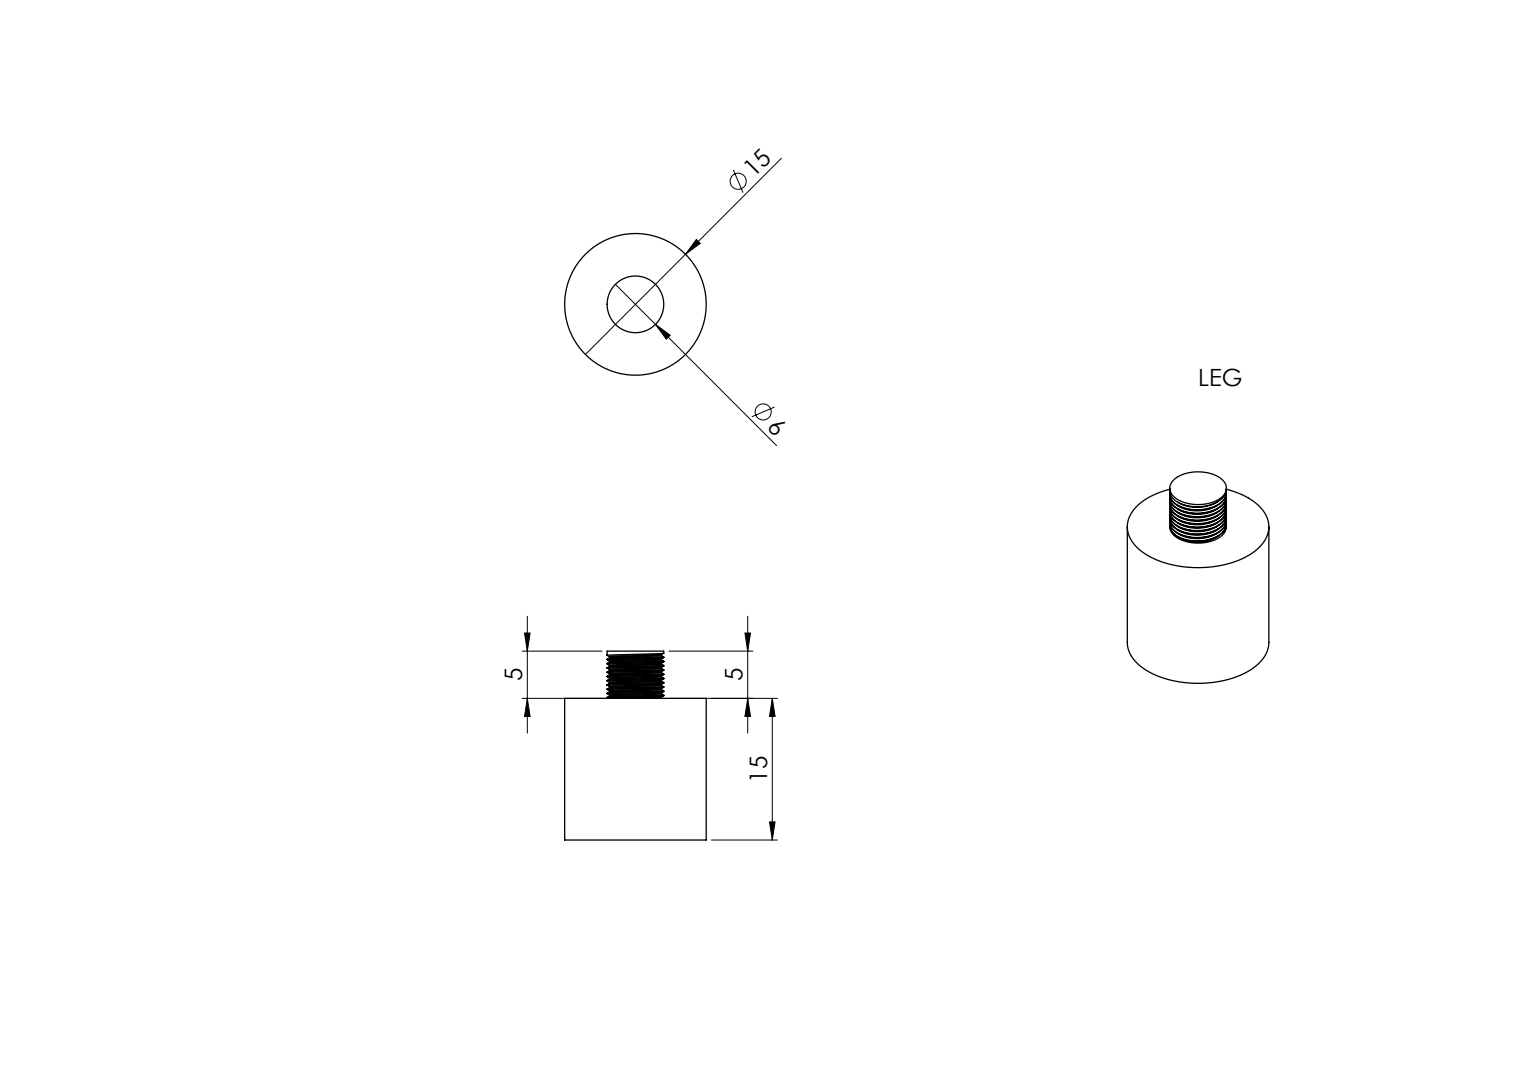
ISO-10303-21;
HEADER;
FILE_DESCRIPTION (('STEP AP214'),
    '1' );
FILE_NAME ('leg.step',
    '2026-10-25T17:17:34',
    ( '' ),
    ( '' ),
    'SwSTEP 2.0',
    'SolidWorks 2026',
    '' );
FILE_SCHEMA (( 'AUTOMOTIVE_DESIGN' ));
ENDSEC;

DATA;
#1=CARTESIAN_POINT ( 'NONE',  ( -79.64356964375001269, -33.59062499938548285, 98.40857419181659793 ) ) ;
#12=CARTESIAN_POINT ( 'NONE',  ( -82.39999999999999147, -34.07812499938548711, 103.1828516163667899 ) ) ;
#16=CARTESIAN_POINT ( 'NONE',  ( -85.39999999999999147, -34.97364041986484295, 98.90809577818235709 ) ) ;
#22=CARTESIAN_POINT ( 'NONE',  ( -79.39999999999999147, -33.41250000000000142, 101.7320508075688537 ) ) ;
#23=CARTESIAN_POINT ( 'NONE',  ( -83.90000000000000568, -30.46874999877096712, 97.40192378864668399 ) ) ;
#27=EDGE_CURVE ( 'NONE', #9630, #12897, #3914, .T. ) ;
#34=CARTESIAN_POINT ( 'NONE',  ( -85.15643035624999868, -31.00312499938548072, 101.5914258081833879 ) ) ;
#40=CARTESIAN_POINT ( 'NONE',  ( -85.40000000000000568, -31.38749999999999574, 98.26794919243111792 ) ) ;
#54=EDGE_CURVE ( 'NONE', #12568, #18235, #14634, .T. ) ;
#61=CARTESIAN_POINT ( 'NONE',  ( -79.39999999999999147, -31.03124999877097068, 98.26794919243110371 ) ) ;
#63=CARTESIAN_POINT ( 'NONE',  ( -85.40000000000000568, -31.38356250001228531, 98.26794919243111792 ) ) ;
#67=CARTESIAN_POINT ( 'NONE',  ( -85.15643035624999868, -31.97812499938548925, 98.40857419181659793 ) ) ;
#73=DIRECTION ( 'NONE',  ( -0.000000000000000000, -1.000000000000000000, -0.000000000000000000 ) ) ;
#93=CARTESIAN_POINT ( 'NONE',  ( -79.39999999999999147, -32.91018749875867400, 101.7320508075688537 ) ) ;
#95=CARTESIAN_POINT ( 'NONE',  ( -82.39999999999999147, -34.19062499938548427, 103.1828516163667899 ) ) ;
#109=CARTESIAN_POINT ( 'NONE',  ( -79.64356964374998427, -33.10312499938548569, 101.5914258081833879 ) ) ;
#112=ORIENTED_EDGE ( 'NONE', *, *, #10203, .F. ) ;
#115=CARTESIAN_POINT ( 'NONE',  ( -82.39999999999999147, -34.83749999999999858, 103.0000000000000000 ) ) ;
#121=CARTESIAN_POINT ( 'NONE',  ( -83.90000000000000568, -34.57500000000000284, 97.40192378864668399 ) ) ;
#122=CARTESIAN_POINT ( 'NONE',  ( -79.39999999999999147, -31.93124999877096926, 98.26794919243110371 ) ) ;
#132=CARTESIAN_POINT ( 'NONE',  ( -82.65380294351676582, -34.99990492518305274, 97.01075526832239859 ) ) ;
#135=CARTESIAN_POINT ( 'NONE',  ( -81.02178482187500208, -31.19062499938548427, 97.61286128772489690 ) ) ;
#141=CARTESIAN_POINT ( 'NONE',  ( -79.39999999999999147, -30.26249999999999929, 101.7320508075688537 ) ) ;
#149=ORIENTED_EDGE ( 'NONE', *, *, #9637, .F. ) ;
#160=CARTESIAN_POINT ( 'NONE',  ( -79.39999999999999147, -32.43356250001229313, 98.26794919243110371 ) ) ;
#189=CARTESIAN_POINT ( 'NONE',  ( -80.90000000000000568, -32.49768749875867968, 102.5980762113533018 ) ) ;
#190=CARTESIAN_POINT ( 'NONE',  ( -83.77821517812500929, -33.02812499938548285, 97.61286128772489690 ) ) ;
#203=CARTESIAN_POINT ( 'NONE',  ( -83.77821517812500929, -33.36562499938548854, 97.61286128772489690 ) ) ;
#204=EDGE_LOOP ( 'NONE', ( #12601, #4330, #15037, #10087 ) ) ;
#212=CARTESIAN_POINT ( 'NONE',  ( -85.40000000000000568, -30.35045094645306563, 101.9998975609119469 ) ) ;
#213=CARTESIAN_POINT ( 'NONE',  ( -82.39999999999999147, -30.73124999877096641, 103.4641016151377499 ) ) ;
#216=CARTESIAN_POINT ( 'NONE',  ( -82.39999999999999147, -35.09062499938548285, 103.1828516163667899 ) ) ;
#222=ORIENTED_EDGE ( 'NONE', *, *, #5417, .T. ) ;
#233=CARTESIAN_POINT ( 'NONE',  ( -83.90000000000000568, -30.07499999999999929, 97.40192378864668399 ) ) ;
#245=CARTESIAN_POINT ( 'NONE',  ( -80.90000000000000568, -31.59374999877097423, 102.5980762113533018 ) ) ;
#248=STYLED_ITEM ( 'NONE', ( #13866 ), #18578 ) ;
#250=CARTESIAN_POINT ( 'NONE',  ( -83.77821517812500929, -31.52812499938548996, 102.3871387122750889 ) ) ;
#254=CARTESIAN_POINT ( 'NONE',  ( -82.31848699153323423, -34.99951142137499716, 103.0191144166183221 ) ) ;
#259=CARTESIAN_POINT ( 'NONE',  ( -85.40000000000000568, -34.96970290221972277, 98.90809659374338025 ) ) ;
#262=CARTESIAN_POINT ( 'NONE',  ( -79.64356964374998427, -30.51562499938548711, 101.5914258081833879 ) ) ;
#276=VECTOR ( 'NONE', #14347, 1000.000000000000000 ) ;
#286=CARTESIAN_POINT ( 'NONE',  ( -79.39999999999999147, -31.52268749875867471, 99.99999999999998579 ) ) ;
#288=CARTESIAN_POINT ( 'NONE',  ( -82.39999999999999147, -33.74062499938548854, 103.1828516163667899 ) ) ;
#304=CARTESIAN_POINT ( 'NONE',  ( -85.15643035625001289, -35.05312499938548143, 101.5914258081833879 ) ) ;
#314=CARTESIAN_POINT ( 'NONE',  ( -79.39999999999999147, -33.78750000000000142, 98.26794919243110371 ) ) ;
#316=CARTESIAN_POINT ( 'NONE',  ( -83.90000000000000568, -30.91874999877096997, 97.40192378864668399 ) ) ;
#319=CARTESIAN_POINT ( 'NONE',  ( -79.39999999999999147, -30.71250000000000213, 101.7320508075688537 ) ) ;
#322=CARTESIAN_POINT ( 'NONE',  ( -82.40000000000000568, -30.00000000000000355, 103.0000000000000000 ) ) ;
#327=FILL_AREA_STYLE ('',( #7917 ) ) ;
#329=DIRECTION ( 'NONE',  ( -0.000000000000000000, -1.000000000000000000, -0.000000000000000000 ) ) ;
#353=CARTESIAN_POINT ( 'NONE',  ( -83.77821517812500929, -30.32812499938548711, 97.61286128772489690 ) ) ;
#357=CARTESIAN_POINT ( 'NONE',  ( -79.76502430829106061, -35.00019033771674515, 98.52379045060148144 ) ) ;
#361=CARTESIAN_POINT ( 'NONE',  ( -83.77821517812500929, -31.07812499938548711, 102.3871387122750889 ) ) ;
#371=CARTESIAN_POINT ( 'NONE',  ( -85.40000000000000568, -33.18750000000000000, 98.26794919243111792 ) ) ;
#380=CARTESIAN_POINT ( 'NONE',  ( -80.90000000000000568, -35.19768749875867542, 102.5980762113533018 ) ) ;
#408=CARTESIAN_POINT ( 'NONE',  ( -82.40000000000000568, -33.93750000000000711, 102.9999999999999858 ) ) ;
#409=CARTESIAN_POINT ( 'NONE',  ( -82.39999999999999147, -30.95624999877097139, 96.53589838486223584 ) ) ;
#410=CARTESIAN_POINT ( 'NONE',  ( -80.90000000000000568, -34.14374999877097139, 97.40192378864668399 ) ) ;
#414=CARTESIAN_POINT ( 'NONE',  ( -85.15643035625001289, -35.22676544108147567, 98.99674642581742035 ) ) ;
#418=ORIENTED_EDGE ( 'NONE', *, *, #10898, .T. ) ;
#441=ORIENTED_EDGE ( 'NONE', *, *, #8685, .F. ) ;
#446=CARTESIAN_POINT ( 'NONE',  ( -79.64356964375001269, -32.24062499938548854, 98.40857419181659793 ) ) ;
#450=CARTESIAN_POINT ( 'NONE',  ( -84.70833260042415702, -35.00006955123599539, 98.08383195543535749 ) ) ;
#454=CARTESIAN_POINT ( 'NONE',  ( -83.77821517812500929, -30.62812499938548783, 102.3871387122750889 ) ) ;
#467=DIRECTION ( 'NONE',  ( 0.000000000000000000, 0.000000000000000000, -1.000000000000000000 ) ) ;
#475=CARTESIAN_POINT ( 'NONE',  ( -85.40000000000000568, -34.03518749875867400, 98.26794919243111792 ) ) ;
#488=CARTESIAN_POINT ( 'NONE',  ( -82.39999999999999147, -33.85312499938547859, 96.81714838363319586 ) ) ;
#500=CARTESIAN_POINT ( 'NONE',  ( -82.39999999999999147, -31.40624999877097068, 96.53589838486223584 ) ) ;
#501=CARTESIAN_POINT ( 'NONE',  ( -82.39999999999999147, -33.20624999877097139, 96.53589838486223584 ) ) ;
#502=CARTESIAN_POINT ( 'NONE',  ( -82.40000000000000568, -30.50624999877097210, 96.99999999999998579 ) ) ;
#521=CARTESIAN_POINT ( 'NONE',  ( -85.40000000000000568, -30.39374999877097139, 99.99999999999998579 ) ) ;
#536=CARTESIAN_POINT ( 'NONE',  ( -79.64356964375001269, -31.41562499938548569, 101.5914258081833879 ) ) ;
#546=CARTESIAN_POINT ( 'NONE',  ( -83.77821517812500929, -32.57812499938548711, 97.61286128772489690 ) ) ;
#555=EDGE_CURVE ( 'NONE', #2812, #11515, #13893, .T. ) ;
#571=CARTESIAN_POINT ( 'NONE',  ( -80.90000000000000568, -34.74768749875867968, 102.5980762113533018 ) ) ;
#580=AXIS2_PLACEMENT_3D ( 'NONE', #9951, #8566, #14520 ) ;
#589=CARTESIAN_POINT ( 'NONE',  ( -83.77821517812500929, -32.31562499938548427, 102.3871387122750889 ) ) ;
#601=CARTESIAN_POINT ( 'NONE',  ( -82.40000000000001990, -32.13750000000000284, 103.0000000000000000 ) ) ;
#602=CARTESIAN_POINT ( 'NONE',  ( -85.40000000000000568, -31.33124999877096428, 98.26794919243111792 ) ) ;
#604=CARTESIAN_POINT ( 'NONE',  ( -79.39999999999999147, -35.11874999877096570, 99.99999999999998579 ) ) ;
#607=CARTESIAN_POINT ( 'NONE',  ( -82.40000000000000568, -30.50624999877097210, 96.99999999999998579 ) ) ;
#612=ORIENTED_EDGE ( 'NONE', *, *, #5825, .F. ) ;
#613=CARTESIAN_POINT ( 'NONE',  ( -83.90000000000000568, -33.46874999877096712, 102.5980762113533018 ) ) ;
#616=CYLINDRICAL_SURFACE ( 'NONE', #18162, 3.000000000000002665 ) ;
#619=CARTESIAN_POINT ( 'NONE',  ( -81.59615242270665192, -33.86115380933864571, 103.0000000000000000 ) ) ;
#625=CARTESIAN_POINT ( 'NONE',  ( -79.39999999999999147, -33.82106250001229597, 99.99999999999998579 ) ) ;
#632=EDGE_LOOP ( 'NONE', ( #11535, #18764, #13842, #12752 ) ) ;
#636=CARTESIAN_POINT ( 'NONE',  ( -83.20384757729335945, -30.80759618943233846, 102.9999999999999858 ) ) ;
#638=CARTESIAN_POINT ( 'NONE',  ( -83.77821517812500929, -31.97812499938548925, 102.3871387122750889 ) ) ;
#647=CARTESIAN_POINT ( 'NONE',  ( -81.02178482187500208, -31.30312499938548498, 97.61286128772489690 ) ) ;
#650=ADVANCED_FACE ( 'NONE', ( #8903 ), #14768, .T. ) ;
#667=ADVANCED_FACE ( 'NONE', ( #13111 ), #7348, .T. ) ;
#669=CARTESIAN_POINT ( 'NONE',  ( -79.39999999999999147, -34.71018749875867826, 101.7320508075688537 ) ) ;
#683=CARTESIAN_POINT ( 'NONE',  ( -83.77821517812500929, -34.56562499938548427, 102.3871387122750889 ) ) ;
#689=ORIENTED_EDGE ( 'NONE', *, *, #8646, .T. ) ;
#693=CARTESIAN_POINT ( 'NONE',  ( -79.39999999999999147, -34.31250000000000000, 101.7320508075688537 ) ) ;
#694=CARTESIAN_POINT ( 'NONE',  ( -79.39999999999999147, -32.90624999877096712, 101.7320508075688537 ) ) ;
#696=CARTESIAN_POINT ( 'NONE',  ( -85.40000000000000568, -34.03124999877096712, 98.26794919243111792 ) ) ;
#697=CARTESIAN_POINT ( 'NONE',  ( -83.90000000000000568, -32.17500000000000426, 102.5980762113533018 ) ) ;
#706=LINE ( 'NONE', #16822, #18035 ) ;
#710=CARTESIAN_POINT ( 'NONE',  ( -82.40000000000000568, -35.00000000000000000, 99.99999999999998579 ) ) ;
#712=CARTESIAN_POINT ( 'NONE',  ( -79.39999999999999147, -31.93124999877096926, 98.26794919243110371 ) ) ;
#714=CARTESIAN_POINT ( 'NONE',  ( -82.40000000000001990, -33.88124999877096855, 103.0000000000000000 ) ) ;
#716=( BOUNDED_CURVE ( )  B_SPLINE_CURVE ( 2, ( #8573, #10335, #8671, #13360, #14625, #1549, #11516, #4377, #5749 ),
 .UNSPECIFIED., .F., .F. ) 
 B_SPLINE_CURVE_WITH_KNOTS ( ( 3, 2, 2, 2, 3 ),
 ( 0.3125000000000001665, 0.3194444444444444198, 0.3333333333333333148, 0.3472222222222222099, 0.3541666666666666297 ),
 .UNSPECIFIED. ) 
 CURVE ( )  GEOMETRIC_REPRESENTATION_ITEM ( )  RATIONAL_B_SPLINE_CURVE ( ( 0.9330127018922194093, 0.9330127018922209636, 1.000000000000000000, 0.8660254037844387076, 1.000000000000000000, 0.8660254037844387076, 1.000000000000000000, 0.9330127018922196314, 0.9330127018922194093 ) ) 
 REPRESENTATION_ITEM ( '' )  );
#718=DIRECTION ( 'NONE',  ( -0.000000000000000000, -1.000000000000000000, -0.000000000000000000 ) ) ;
#720=CARTESIAN_POINT ( 'NONE',  ( -80.90000000000000568, -30.30000000000000426, 102.5980762113533018 ) ) ;
#724=DIRECTION ( 'NONE',  ( -0.000000000000000000, -1.000000000000000000, -0.000000000000000000 ) ) ;
#733=CARTESIAN_POINT ( 'NONE',  ( -82.39999999999999147, -33.06562499938548427, 96.81714838363319586 ) ) ;
#740=CARTESIAN_POINT ( 'NONE',  ( -81.02178482187500208, -32.65312499938548996, 97.61286128772489690 ) ) ;
#750=CARTESIAN_POINT ( 'NONE',  ( -83.20384757729335945, -33.00134618820329990, 102.9999999999999858 ) ) ;
#762=CARTESIAN_POINT ( 'NONE',  ( -79.39999999999999147, -33.36018749875868394, 101.7320508075688537 ) ) ;
#765=DIRECTION ( 'NONE',  ( 0.000000000000000000, -0.000000000000000000, 1.000000000000000000 ) ) ;
#767=FACE_OUTER_BOUND ( 'NONE', #5223, .T. ) ;
#776=CARTESIAN_POINT ( 'NONE',  ( -79.64356964374999848, -33.51562499938548711, 99.99999999999998579 ) ) ;
#788=CARTESIAN_POINT ( 'NONE',  ( -85.40000000000000568, -31.70624999877096784, 101.7320508075688679 ) ) ;
#789=CARTESIAN_POINT ( 'NONE',  ( -85.40000000000000568, -33.09374999877096712, 99.99999999999998579 ) ) ;
#805=CARTESIAN_POINT ( 'NONE',  ( -85.15643035625001289, -30.25312499938548783, 99.99999999999998579 ) ) ;
#806=STYLED_ITEM('',(#19357),#9467);
#811=CARTESIAN_POINT ( 'NONE',  ( -83.20384757729337366, -30.48615380933863150, 97.00000000000000000 ) ) ;
#813=CARTESIAN_POINT ( 'NONE',  ( -79.39999999999999147, -30.63750000000000284, 98.26794919243110371 ) ) ;
#828=CARTESIAN_POINT ( 'NONE',  ( -79.64356964375001269, -34.49062499938548854, 98.40857419181659793 ) ) ;
#837=CARTESIAN_POINT ( 'NONE',  ( -82.39999999999999147, -33.51562499938548711, 96.81714838363319586 ) ) ;
#846=CARTESIAN_POINT ( 'NONE',  ( -80.90000000000000568, -34.35000000000000853, 102.5980762113533018 ) ) ;
#853=CYLINDRICAL_SURFACE ( 'NONE', #4855, 3.000000000000002665 ) ;
#854=CARTESIAN_POINT ( 'NONE',  ( -85.40000000000000568, -30.48356250001229029, 98.26794919243111792 ) ) ;
#873=CARTESIAN_POINT ( 'NONE',  ( -79.64356964375001269, -33.10312499938549280, 101.5914258081833879 ) ) ;
#877=FACE_OUTER_BOUND ( 'NONE', #6470, .T. ) ;
#884=CARTESIAN_POINT ( 'NONE',  ( -82.39999999999999147, -31.63124999877097210, 103.4641016151377499 ) ) ;
#885=CARTESIAN_POINT ( 'NONE',  ( -85.40000000000000568, -35.36739044046696279, 98.90809476984486537 ) ) ;
#886=VECTOR ( 'NONE', #2876, 1000.000000000000000 ) ;
#897=ORIENTED_EDGE ( 'NONE', *, *, #8064, .F. ) ;
#899=CARTESIAN_POINT ( 'NONE',  ( -82.39999999999999147, -30.47812499938548569, 103.1828516163667899 ) ) ;
#905=ADVANCED_FACE ( 'NONE', ( #18104, #4715 ), #15646, .F. ) ;
#910=CARTESIAN_POINT ( 'NONE',  ( -83.90000000000000568, -33.97106250001230165, 102.5980762113533018 ) ) ;
#915=CYLINDRICAL_SURFACE ( 'NONE', #17436, 3.000000000000002665 ) ;
#917=( BOUNDED_CURVE ( )  B_SPLINE_CURVE ( 2, ( #8964, #4479, #7598, #11995, #3006, #16396, #4288, #14932, #1556 ),
 .UNSPECIFIED., .F., .F. ) 
 B_SPLINE_CURVE_WITH_KNOTS ( ( 3, 2, 2, 2, 3 ),
 ( 0.2708333333333333148, 0.2777777777777777901, 0.2916666666666666852, 0.3055555555555555802, 0.3125000000000001110 ),
 .UNSPECIFIED. ) 
 CURVE ( )  GEOMETRIC_REPRESENTATION_ITEM ( )  RATIONAL_B_SPLINE_CURVE ( ( 0.9330127018922194093, 0.9330127018922190762, 1.000000000000000000, 0.8660254037844387076, 1.000000000000000000, 0.8660254037844387076, 1.000000000000000000, 0.9330127018922182991, 0.9330127018922194093 ) ) 
 REPRESENTATION_ITEM ( '' )  );
#919=ORIENTED_EDGE ( 'NONE', *, *, #16886, .F. ) ;
#924=CARTESIAN_POINT ( 'NONE',  ( -79.64356964375001269, -35.01562499938548711, 101.5914258081833879 ) ) ;
#928=CARTESIAN_POINT ( 'NONE',  ( -82.30067660862302148, -35.00052948526250418, 96.98128288508057437 ) ) ;
#929=CARTESIAN_POINT ( 'NONE',  ( -85.15643035624999868, -34.67812499938548143, 98.40857419181659793 ) ) ;
#930=CARTESIAN_POINT ( 'NONE',  ( -82.40000000000000568, -35.00000000000000000, 107.5000000000000142 ) ) ;
#934=ADVANCED_FACE ( 'NONE', ( #12608 ), #616, .T. ) ;
#935=CARTESIAN_POINT ( 'NONE',  ( -79.64356964374998427, -34.56562499938548427, 101.5914258081833879 ) ) ;
#946=CARTESIAN_POINT ( 'NONE',  ( -80.90000000000000568, -33.45000000000000284, 102.5980762113533018 ) ) ;
#950=CARTESIAN_POINT ( 'NONE',  ( -83.90000000000000568, -31.42500000000000071, 97.40192378864668399 ) ) ;
#954=CARTESIAN_POINT ( 'NONE',  ( -82.40000000000000568, -30.00000000000000355, 99.99999999999998579 ) ) ;
#956=CARTESIAN_POINT ( 'NONE',  ( -85.40000000000000568, -30.93356250001229313, 98.26794919243111792 ) ) ;
#957=CYLINDRICAL_SURFACE ( 'NONE', #2043, 3.000000000000002665 ) ;
#959=CARTESIAN_POINT ( 'NONE',  ( -85.15643035625001289, -30.59062499938548285, 99.99999999999998579 ) ) ;
#960=DIRECTION ( 'NONE',  ( 0.000000000000000000, 0.000000000000000000, -1.000000000000000000 ) ) ;
#980=CARTESIAN_POINT ( 'NONE',  ( -80.90000000000000568, -34.74374999877097281, 102.5980762113533018 ) ) ;
#981=CARTESIAN_POINT ( 'NONE',  ( -85.15643035624999868, -31.56562499938548427, 101.5914258081833879 ) ) ;
#991=CARTESIAN_POINT ( 'NONE',  ( -83.90000000000000568, -35.26874999877097139, 102.5980762113533018 ) ) ;
#997=ORIENTED_EDGE ( 'NONE', *, *, #5541, .F. ) ;
#1004=CARTESIAN_POINT ( 'NONE',  ( -80.90000000000000568, -32.85000000000000142, 97.40192378864668399 ) ) ;
#1013=CARTESIAN_POINT ( 'NONE',  ( -82.40000000000000568, -30.00000000000000355, 96.99999999999998579 ) ) ;
#1019=CARTESIAN_POINT ( 'NONE',  ( -82.39999999999999147, -33.74062499938548854, 103.1828516163667899 ) ) ;
#1023=CARTESIAN_POINT ( 'NONE',  ( -83.77821517812500929, -34.26562499938548711, 97.61286128772489690 ) ) ;
#1028=CARTESIAN_POINT ( 'NONE',  ( -83.77821517812500929, -33.02812499938548285, 97.61286128772489690 ) ) ;
#1038=CARTESIAN_POINT ( 'NONE',  ( -83.90000000000000568, -33.22500000000000142, 97.40192378864668399 ) ) ;
#1039=AXIS2_PLACEMENT_3D ( 'NONE', #9542, #18538, #13936 ) ;
#1050=CARTESIAN_POINT ( 'NONE',  ( -79.64356964375001269, -30.32812499938548711, 98.40857419181659793 ) ) ;
#1059=CARTESIAN_POINT ( 'NONE',  ( -81.02178482187500208, -34.79062499938548569, 97.61286128772489690 ) ) ;
#1069=CARTESIAN_POINT ( 'NONE',  ( -82.39999999999999147, -35.23124999877096997, 103.4641016151377499 ) ) ;
#1070=CARTESIAN_POINT ( 'NONE',  ( -85.40000000000000568, -35.34374999877096712, 99.99999999999998579 ) ) ;
#1081=CARTESIAN_POINT ( 'NONE',  ( -85.15643035625001289, -31.49062499938548498, 99.99999999999998579 ) ) ;
#1089=CARTESIAN_POINT ( 'NONE',  ( -79.39999999999999147, -31.61250000000000071, 101.7320508075688537 ) ) ;
#1095=CARTESIAN_POINT ( 'NONE',  ( -79.39999999999999147, -31.08750000000000568, 98.26794919243110371 ) ) ;
#1102=CARTESIAN_POINT ( 'NONE',  ( -79.64356964375001269, -34.04062499938549280, 98.40857419181659793 ) ) ;
#1106=CARTESIAN_POINT ( 'NONE',  ( -82.39999999999999147, -33.85312499938547859, 96.81714838363319586 ) ) ;
#1114=CARTESIAN_POINT ( 'NONE',  ( -83.77821517812500929, -33.92812499938548854, 97.61286128772489690 ) ) ;
#1126=CARTESIAN_POINT ( 'NONE',  ( -80.90000000000000568, -34.20000000000000284, 97.40192378864668399 ) ) ;
#1148=ORIENTED_EDGE ( 'NONE', *, *, #9637, .T. ) ;
#1155=VERTEX_POINT ( 'NONE', #12694 ) ;
#1164=CARTESIAN_POINT ( 'NONE',  ( -83.90000000000000568, -33.61874999877097281, 97.40192378864668399 ) ) ;
#1166=CARTESIAN_POINT ( 'NONE',  ( -79.64356964374999848, -30.92812499938548498, 99.99999999999998579 ) ) ;
#1179=CARTESIAN_POINT ( 'NONE',  ( -79.64356964374998427, -31.30312499938548143, 101.5914258081833879 ) ) ;
#1180=VECTOR ( 'NONE', #3831, 1000.000000000000000 ) ;
#1187=CARTESIAN_POINT ( 'NONE',  ( -85.40000000000000568, -31.74374999877096926, 99.99999999999998579 ) ) ;
#1190=VECTOR ( 'NONE', #1364, 1000.000000000000000 ) ;
#1193=CARTESIAN_POINT ( 'NONE',  ( -82.39999999999999147, -32.13749999999999574, 103.4641016151377499 ) ) ;
#1202=CARTESIAN_POINT ( 'NONE',  ( -80.90000000000000568, -33.39374999877097139, 102.5980762113533018 ) ) ;
#1204=CARTESIAN_POINT ( 'NONE',  ( -82.39999999999999147, -31.60312499938548569, 96.81714838363319586 ) ) ;
#1208=CARTESIAN_POINT ( 'NONE',  ( -85.15643035624999868, -33.32812499938548001, 98.40857419181659793 ) ) ;
#1211=CARTESIAN_POINT ( 'NONE',  ( -82.40000000000000568, -30.00000000000000355, 103.0000000000000000 ) ) ;
#1215=CARTESIAN_POINT ( 'NONE',  ( -81.02178482187500208, -35.05312499938548854, 102.3871387122750889 ) ) ;
#1222=EDGE_LOOP ( 'NONE', ( #8619, #10140 ) ) ;
#1224=CARTESIAN_POINT ( 'NONE',  ( -82.40000000000000568, -30.00000000000000355, 99.99999999999998579 ) ) ;
#1226=CARTESIAN_POINT ( 'NONE',  ( -79.39999999999999147, -32.88750000000000284, 98.26794919243110371 ) ) ;
#1236=CARTESIAN_POINT ( 'NONE',  ( -82.40000000000000568, -30.00000000000000355, 96.99999999999998579 ) ) ;
#1238=CARTESIAN_POINT ( 'NONE',  ( -83.77821517812500929, -32.01562499938548001, 97.61286128772489690 ) ) ;
#1254=ORIENTED_EDGE ( 'NONE', *, *, #2671, .T. ) ;
#1265=CARTESIAN_POINT ( 'NONE',  ( -79.39999999999999147, -35.11874999877096570, 99.99999999999998579 ) ) ;
#1266=CARTESIAN_POINT ( 'NONE',  ( -81.02178482187500208, -31.75312499938548427, 97.61286128772489690 ) ) ;
#1272=VERTEX_POINT ( 'NONE', #607 ) ;
#1277=CARTESIAN_POINT ( 'NONE',  ( -83.77821517812500929, -32.91562499938547859, 97.61286128772489690 ) ) ;
#1290=CARTESIAN_POINT ( 'NONE',  ( -83.90000000000000568, -33.07500000000000284, 102.5980762113533018 ) ) ;
#1292=DIRECTION ( 'NONE',  ( 0.000000000000000000, 1.000000000000000000, 0.000000000000000000 ) ) ;
#1297=ORIENTED_EDGE ( 'NONE', *, *, #5113, .F. ) ;
#1303=CARTESIAN_POINT ( 'NONE',  ( -83.77821517812500929, -35.12812499938548427, 102.3871387122750889 ) ) ;
#1307=ORIENTED_EDGE ( 'NONE', *, *, #7912, .F. ) ;
#1309=CARTESIAN_POINT ( 'NONE',  ( -82.39999999999999147, -34.97812499938547859, 103.1828516163667899 ) ) ;
#1312=CARTESIAN_POINT ( 'NONE',  ( -83.90000000000000568, -32.62500000000000000, 102.5980762113533018 ) ) ;
#1317=VECTOR ( 'NONE', #9535, 1000.000000000000000 ) ;
#1328=EDGE_CURVE ( 'NONE', #7637, #16985, #16283, .T. ) ;
#1329=AXIS2_PLACEMENT_3D ( 'NONE', #5503, #1292, #12818 ) ;
#1331=( BOUNDED_CURVE ( )  B_SPLINE_CURVE ( 2, ( #6021, #10319, #7768, #12165, #6310, #16373, #13437, #7481, #15187 ),
 .UNSPECIFIED., .F., .F. ) 
 B_SPLINE_CURVE_WITH_KNOTS ( ( 3, 2, 2, 2, 3 ),
 ( 0.5208333333333333703, 0.5277777777777777901, 0.5416666666666666297, 0.5555555555555555802, 0.5625000000000000000 ),
 .UNSPECIFIED. ) 
 CURVE ( )  GEOMETRIC_REPRESENTATION_ITEM ( )  RATIONAL_B_SPLINE_CURVE ( ( 0.9330127018922192983, 0.9330127018922198534, 1.000000000000000000, 0.8660254037844387076, 1.000000000000000000, 0.8660254037844387076, 1.000000000000000000, 0.9330127018922194093, 0.9330127018922194093 ) ) 
 REPRESENTATION_ITEM ( '' )  );
#1334=CARTESIAN_POINT ( 'NONE',  ( -85.40000000000000568, -33.63356250001229597, 98.26794919243111792 ) ) ;
#1337=CARTESIAN_POINT ( 'NONE',  ( -85.15643035625001289, -31.94062499938548427, 99.99999999999998579 ) ) ;
#1361=CARTESIAN_POINT ( 'NONE',  ( -82.39999999999999147, -33.65624999877096712, 96.53589838486223584 ) ) ;
#1362=CARTESIAN_POINT ( 'NONE',  ( -81.02178482187500208, -32.80312499938548854, 102.3871387122750889 ) ) ;
#1364=DIRECTION ( 'NONE',  ( -0.000000000000000000, -1.000000000000000000, -0.000000000000000000 ) ) ;
#1365=ADVANCED_FACE ( 'NONE', ( #3175 ), #10413, .T. ) ;
#1375=CARTESIAN_POINT ( 'NONE',  ( -82.39999999999999147, -32.50312499938548427, 96.81714838363319586 ) ) ;
#1386=CARTESIAN_POINT ( 'NONE',  ( -85.40000000000000568, -32.70000000000000284, 99.99999999999998579 ) ) ;
#1387=CARTESIAN_POINT ( 'NONE',  ( -83.90000000000000568, -31.81874999877096855, 97.40192378864668399 ) ) ;
#1389=CARTESIAN_POINT ( 'NONE',  ( -84.69814161231457206, -35.29583579514545733, 98.07164704222797980 ) ) ;
#1395=CARTESIAN_POINT ( 'NONE',  ( -82.39999999999999147, -30.78750000000000142, 102.9999999999999858 ) ) ;
#1396=CARTESIAN_POINT ( 'NONE',  ( -82.39999999999999147, -30.92812499938548143, 103.1828516163667899 ) ) ;
#1402=CARTESIAN_POINT ( 'NONE',  ( -82.39999999999999147, -32.13749999999999574, 103.4641016151377499 ) ) ;
#1405=CARTESIAN_POINT ( 'NONE',  ( -82.40000000000001990, -31.68750000000000711, 103.0000000000000000 ) ) ;
#1418=( BOUNDED_CURVE ( )  B_SPLINE_CURVE ( 2, ( #15673, #15769, #12741, #7856, #9413, #12539, #15380, #16945, #18611 ),
 .UNSPECIFIED., .F., .F. ) 
 B_SPLINE_CURVE_WITH_KNOTS ( ( 3, 2, 2, 2, 3 ),
 ( 0.7708333333333331483, 0.7777777777777777901, 0.7916666666666666297, 0.8055555555555555802, 0.8125000000000001110 ),
 .UNSPECIFIED. ) 
 CURVE ( )  GEOMETRIC_REPRESENTATION_ITEM ( )  RATIONAL_B_SPLINE_CURVE ( ( 0.9330127018922194093, 0.9330127018922177440, 1.000000000000000000, 0.8660254037844387076, 1.000000000000000000, 0.8660254037844387076, 1.000000000000000000, 0.9330127018922182991, 0.9330127018922194093 ) ) 
 REPRESENTATION_ITEM ( '' )  );
#1424=CARTESIAN_POINT ( 'NONE',  ( -80.90000000000000568, -32.39606250001229881, 97.40192378864668399 ) ) ;
#1427=CARTESIAN_POINT ( 'NONE',  ( -79.64356964374999848, -32.16562499938548569, 99.99999999999998579 ) ) ;
#1450=CARTESIAN_POINT ( 'NONE',  ( -80.90000000000000568, -31.59768749875868110, 102.5980762113533018 ) ) ;
#1451=CARTESIAN_POINT ( 'NONE',  ( -85.15643035625001289, -32.50312499938548427, 99.99999999999998579 ) ) ;
#1455=CARTESIAN_POINT ( 'NONE',  ( -84.51155153715826884, -35.14114847181267720, 98.22820474807231506 ) ) ;
#1463=CARTESIAN_POINT ( 'NONE',  ( -82.39999999999999147, -33.85312499938548569, 96.81714838363319586 ) ) ;
#1474=CARTESIAN_POINT ( 'NONE',  ( -80.90000000000000568, -30.69374999877097210, 102.5980762113533018 ) ) ;
#1475=CARTESIAN_POINT ( 'NONE',  ( -82.39999999999999147, -30.50624999877097210, 96.53589838486223584 ) ) ;
#1491=CARTESIAN_POINT ( 'NONE',  ( -79.64356964375001269, -32.20312499938548001, 101.5914258081833879 ) ) ;
#1492=DIRECTION ( 'NONE',  ( 0.000000000000000000, -1.000000000000000000, 0.000000000000000000 ) ) ;
#1496=ORIENTED_EDGE ( 'NONE', *, *, #6126, .T. ) ;
#1499=CARTESIAN_POINT ( 'NONE',  ( -85.40000000000000568, -32.25000000000000000, 99.99999999999998579 ) ) ;
#1511=EDGE_CURVE ( 'NONE', #2507, #16323, #4665, .T. ) ;
#1524=CARTESIAN_POINT ( 'NONE',  ( -82.40000000000000568, -30.95624999877097139, 96.99999999999998579 ) ) ;
#1526=CARTESIAN_POINT ( 'NONE',  ( -83.90000000000000568, -32.77106250001229171, 97.40192378864668399 ) ) ;
#1530=CARTESIAN_POINT ( 'NONE',  ( -79.64356964375001269, -30.85312499938548569, 101.5914258081833879 ) ) ;
#1535=DIRECTION ( 'NONE',  ( 0.000000000000000000, 0.000000000000000000, -1.000000000000000000 ) ) ;
#1538=( BOUNDED_CURVE ( )  B_SPLINE_CURVE ( 2, ( #16992, #4802, #3314, #13857, #15532, #12495, #13768, #9271, #408 ),
 .UNSPECIFIED., .F., .F. ) 
 B_SPLINE_CURVE_WITH_KNOTS ( ( 3, 2, 2, 2, 3 ),
 ( 0.6875000000000000000, 0.6944444444444444198, 0.7083333333333333703, 0.7222222222222222099, 0.7291666666666668517 ),
 .UNSPECIFIED. ) 
 CURVE ( )  GEOMETRIC_REPRESENTATION_ITEM ( )  RATIONAL_B_SPLINE_CURVE ( ( 0.9330127018922194093, 0.9330127018922194093, 1.000000000000000000, 0.8660254037844387076, 1.000000000000000000, 0.8660254037844387076, 1.000000000000000000, 0.9330127018922177440, 0.9330127018922194093 ) ) 
 REPRESENTATION_ITEM ( '' )  );
#1549=CARTESIAN_POINT ( 'NONE',  ( -85.40000000000000568, -32.23124999877096997, 98.26794919243111792 ) ) ;
#1554=CARTESIAN_POINT ( 'NONE',  ( -79.39999999999999147, -31.48518749875868394, 98.26794919243110371 ) ) ;
#1555=CARTESIAN_POINT ( 'NONE',  ( -83.77821517812500929, -32.87812499938548427, 102.3871387122750889 ) ) ;
#1556=CARTESIAN_POINT ( 'NONE',  ( -82.40000000000000568, -31.68750000000000711, 102.9999999999999858 ) ) ;
#1567=CARTESIAN_POINT ( 'NONE',  ( -81.02178482187500208, -34.49062499938548854, 102.3871387122750889 ) ) ;
#1571=CARTESIAN_POINT ( 'NONE',  ( -82.40000000000000568, -34.10624999877096997, 96.99999999999998579 ) ) ;
#1577=CARTESIAN_POINT ( 'NONE',  ( -79.39999999999999147, -34.68750000000000000, 98.26794919243110371 ) ) ;
#1578=CARTESIAN_POINT ( 'NONE',  ( -79.39999999999999147, -32.41874999877096997, 99.99999999999998579 ) ) ;
#1589=CARTESIAN_POINT ( 'NONE',  ( -82.39999999999999147, -31.15312499938548640, 96.81714838363319586 ) ) ;
#1595=ORIENTED_EDGE ( 'NONE', *, *, #7912, .T. ) ;
#1597=CARTESIAN_POINT ( 'NONE',  ( -85.40000000000000568, -30.86250000000000071, 101.7320508075688679 ) ) ;
#1612=CARTESIAN_POINT ( 'NONE',  ( -83.32052461991715120, -34.98323688327303671, 97.06736352196708140 ) ) ;
#1615=ORIENTED_EDGE ( 'NONE', *, *, #11751, .T. ) ;
#1619=CARTESIAN_POINT ( 'NONE',  ( -85.40000000000000568, -31.83356250001229881, 98.26794919243111792 ) ) ;
#1625=DIRECTION ( 'NONE',  ( 0.000000000000000000, 0.000000000000000000, -1.000000000000000000 ) ) ;
#1627=ORIENTED_EDGE ( 'NONE', *, *, #11751, .F. ) ;
#1643=CARTESIAN_POINT ( 'NONE',  ( -83.90000000000000568, -33.02268749875867826, 102.5980762113533018 ) ) ;
#1644=CARTESIAN_POINT ( 'NONE',  ( -79.64356964374999848, -33.17812499938548854, 99.99999999999998579 ) ) ;
#1658=CARTESIAN_POINT ( 'NONE',  ( -85.15643035625001289, -33.29062499938547859, 99.99999999999998579 ) ) ;
#1663=CARTESIAN_POINT ( 'NONE',  ( -85.40000000000000568, -34.95000000000000284, 99.99999999999998579 ) ) ;
#1669=CARTESIAN_POINT ( 'NONE',  ( -85.40000000000000568, -34.05000000000000426, 99.99999999999998579 ) ) ;
#1670=CARTESIAN_POINT ( 'NONE',  ( -83.90000000000000568, -32.71874999877096712, 97.40192378864668399 ) ) ;
#1671=CARTESIAN_POINT ( 'NONE',  ( -82.40000000000000568, -30.00000000000000355, 99.99999999999998579 ) ) ;
#1687=CARTESIAN_POINT ( 'NONE',  ( -79.39999999999999147, -30.18750000000000355, 98.26794919243110371 ) ) ;
#1704=CARTESIAN_POINT ( 'NONE',  ( -84.94178044275902550, -34.99917348188823496, 101.6311593377337203 ) ) ;
#1707=CARTESIAN_POINT ( 'NONE',  ( -80.90000000000000568, -33.29606250001229739, 97.40192378864668399 ) ) ;
#1709=CARTESIAN_POINT ( 'NONE',  ( -79.64356964374999848, -31.82812499938548356, 99.99999999999998579 ) ) ;
#1731=CARTESIAN_POINT ( 'NONE',  ( -85.40000000000000568, -31.33518749875867471, 98.26794919243111792 ) ) ;
#1733=CARTESIAN_POINT ( 'NONE',  ( -83.77821517812500929, -33.47812499938548569, 97.61286128772489690 ) ) ;
#1755=DIRECTION ( 'NONE',  ( -0.000000000000000000, -1.000000000000000000, -0.000000000000000000 ) ) ;
#1758=CARTESIAN_POINT ( 'NONE',  ( -79.39999999999999147, -34.31250000000000000, 101.7320508075688537 ) ) ;
#1760=CARTESIAN_POINT ( 'NONE',  ( -80.90000000000000568, -31.44374999877096855, 97.40192378864668399 ) ) ;
#1787=ORIENTED_EDGE ( 'NONE', *, *, #2182, .F. ) ;
#1793=CARTESIAN_POINT ( 'NONE',  ( -81.02178482187500208, -32.20312499938548711, 97.61286128772489690 ) ) ;
#1797=CARTESIAN_POINT ( 'NONE',  ( -79.39923258946704721, -35.00058613678730524, 99.84651357762385260 ) ) ;
#1798=CARTESIAN_POINT ( 'NONE',  ( -80.90000000000000568, -31.14374999877097139, 102.5980762113533018 ) ) ;
#1803=CARTESIAN_POINT ( 'NONE',  ( -85.15643035625001289, -30.66562499938548569, 101.5914258081833879 ) ) ;
#1807=AXIS2_PLACEMENT_3D ( 'NONE', #10995, #6415, #6609 ) ;
#1813=CARTESIAN_POINT ( 'NONE',  ( -83.90000000000000568, -33.01874999877097139, 102.5980762113533018 ) ) ;
#1815=ADVANCED_FACE ( 'NONE', ( #16069 ), #2580, .T. ) ;
#1816=DIRECTION ( 'NONE',  ( 0.000000000000000000, 0.000000000000000000, -1.000000000000000000 ) ) ;
#1819=ORIENTED_EDGE ( 'NONE', *, *, #7074, .F. ) ;
#1828=CARTESIAN_POINT ( 'NONE',  ( -83.90000000000000568, -31.82268749875867542, 97.40192378864668399 ) ) ;
#1845=CARTESIAN_POINT ( 'NONE',  ( -85.15643035625001289, -35.09062499938548285, 99.99999999999998579 ) ) ;
#1846=ORIENTED_EDGE ( 'NONE', *, *, #7551, .F. ) ;
#1855=CARTESIAN_POINT ( 'NONE',  ( -83.90000000000000568, -33.97500000000000853, 102.5980762113533018 ) ) ;
#1856=CARTESIAN_POINT ( 'NONE',  ( -79.39999999999999147, -34.66874999877096997, 99.99999999999998579 ) ) ;
#1857=CARTESIAN_POINT ( 'NONE',  ( -81.59615242270662350, -30.52634618820330914, 97.00000000000000000 ) ) ;
#1858=CARTESIAN_POINT ( 'NONE',  ( -79.39999999999999147, -30.67500000000000071, 99.99999999999998579 ) ) ;
#1863=ORIENTED_EDGE ( 'NONE', *, *, #14991, .T. ) ;
#1864=( NAMED_UNIT ( * ) PLANE_ANGLE_UNIT ( ) SI_UNIT ( $, .RADIAN. ) );
#1889=CARTESIAN_POINT ( 'NONE',  ( -83.90000000000000568, -33.91874999877096997, 102.5980762113533018 ) ) ;
#1891=CARTESIAN_POINT ( 'NONE',  ( -83.77821517812500929, -30.62812499938548783, 102.3871387122750889 ) ) ;
#1895=CARTESIAN_POINT ( 'NONE',  ( -83.35106844018336858, -35.00071516271440686, 102.8502752770200601 ) ) ;
#1897=CARTESIAN_POINT ( 'NONE',  ( -81.59615242270662350, -32.56740381056766864, 103.0000000000000000 ) ) ;
#1899=CARTESIAN_POINT ( 'NONE',  ( -83.77821517812500929, -32.42812499938548854, 102.3871387122750889 ) ) ;
#1919=CARTESIAN_POINT ( 'NONE',  ( -85.40000000000000568, -33.96018749875868536, 101.7320508075688679 ) ) ;
#1936=CARTESIAN_POINT ( 'NONE',  ( -79.64356964375001269, -34.00312499938549138, 101.5914258081833879 ) ) ;
#1949=CARTESIAN_POINT ( 'NONE',  ( -80.90000000000000568, -32.79374999877096997, 97.40192378864668399 ) ) ;
#1950=( BOUNDED_CURVE ( )  B_SPLINE_CURVE ( 2, ( #5196, #14451, #9585, #712, #9979, #17110, #8312, #2349, #4017 ),
 .UNSPECIFIED., .F., .F. ) 
 B_SPLINE_CURVE_WITH_KNOTS ( ( 3, 2, 2, 2, 3 ),
 ( 0.2708333333333333703, 0.2777777777777777901, 0.2916666666666666852, 0.3055555555555555802, 0.3125000000000001665 ),
 .UNSPECIFIED. ) 
 CURVE ( )  GEOMETRIC_REPRESENTATION_ITEM ( )  RATIONAL_B_SPLINE_CURVE ( ( 0.9330127018922194093, 0.9330127018922196314, 1.000000000000000000, 0.8660254037844387076, 1.000000000000000000, 0.8660254037844387076, 1.000000000000000000, 0.9330127018922177440, 0.9330127018922194093 ) ) 
 REPRESENTATION_ITEM ( '' )  );
#1951=CARTESIAN_POINT ( 'NONE',  ( -79.39999999999999147, -33.35624999877097707, 101.7320508075688537 ) ) ;
#1952=CARTESIAN_POINT ( 'NONE',  ( -83.20384757729337366, -32.15759618943233278, 103.0000000000000000 ) ) ;
#1989=CARTESIAN_POINT ( 'NONE',  ( -83.77821517812500929, -31.22812499938548569, 97.61286128772489690 ) ) ;
#1994=CARTESIAN_POINT ( 'NONE',  ( -84.50041942204053669, -34.99839409658486034, 102.1701536479666999 ) ) ;
#1998=CARTESIAN_POINT ( 'NONE',  ( -81.02178482187500208, -30.85312499938548569, 97.61286128772489690 ) ) ;
#2009=CARTESIAN_POINT ( 'NONE',  ( -82.39999999999999147, -33.48750000000000426, 103.0000000000000000 ) ) ;
#2014=CARTESIAN_POINT ( 'NONE',  ( -79.39999999999999147, -32.83124999877097139, 98.26794919243110371 ) ) ;
#2016=CARTESIAN_POINT ( 'NONE',  ( -82.39999999999999147, -34.33518749875868536, 103.4641016151377499 ) ) ;
#2032=CARTESIAN_POINT ( 'NONE',  ( -79.64356964374999848, -33.06562499938548427, 99.99999999999998579 ) ) ;
#2034=VERTEX_POINT ( 'NONE', #18121 ) ;
#2037=CARTESIAN_POINT ( 'NONE',  ( -85.40000000000000568, -30.80624999877096570, 101.7320508075688821 ) ) ;
#2043=AXIS2_PLACEMENT_3D ( 'NONE', #5454, #6912, #18832 ) ;
#2045=CARTESIAN_POINT ( 'NONE',  ( -85.40000000000000568, -33.05624999877096570, 101.7320508075688679 ) ) ;
#2046=CARTESIAN_POINT ( 'NONE',  ( -82.39999999999999147, -35.00624999877097565, 96.53589838486223584 ) ) ;
#2057=CARTESIAN_POINT ( 'NONE',  ( -83.20384757729335945, -33.45134618820330985, 102.9999999999999858 ) ) ;
#2058=CARTESIAN_POINT ( 'NONE',  ( -85.40000000000000568, -30.39374999877097139, 99.99999999999998579 ) ) ;
#2071=CARTESIAN_POINT ( 'NONE',  ( -85.40000000000000568, -34.00856250001229597, 101.7320508075688679 ) ) ;
#2086=CARTESIAN_POINT ( 'NONE',  ( -85.15643035625001289, -30.70312499938548711, 99.99999999999998579 ) ) ;
#2090=ORIENTED_EDGE ( 'NONE', *, *, #7559, .F. ) ;
#2095=CARTESIAN_POINT ( 'NONE',  ( -85.15643035625001289, -30.70312499938548711, 99.99999999999998579 ) ) ;
#2114=AXIS2_PLACEMENT_3D ( 'NONE', #19302, #11861, #16360 ) ;
#2120=CARTESIAN_POINT ( 'NONE',  ( -82.39999999999999147, -34.56018749875867258, 96.53589838486223584 ) ) ;
#2135=SHAPE_DEFINITION_REPRESENTATION ( #13860, #16991 ) ;
#2138=CARTESIAN_POINT ( 'NONE',  ( -79.64356964375001269, -34.45312499938548711, 101.5914258081833879 ) ) ;
#2150=CARTESIAN_POINT ( 'NONE',  ( -79.39999999999999147, -31.48124999877097352, 98.26794919243110371 ) ) ;
#2151=CARTESIAN_POINT ( 'NONE',  ( -85.40000000000000568, -33.50624999877096855, 101.7320508075688679 ) ) ;
#2173=CARTESIAN_POINT ( 'NONE',  ( -82.39999999999999147, -30.11250000000000426, 96.53589838486223584 ) ) ;
#2182=EDGE_CURVE ( 'NONE', #18235, #10587, #17387, .T. ) ;
#2186=CARTESIAN_POINT ( 'NONE',  ( -85.15643035624999868, -30.29062499938548925, 98.40857419181659793 ) ) ;
#2194=CARTESIAN_POINT ( 'NONE',  ( -83.77821517812500929, -34.37812499938548427, 97.61286128772489690 ) ) ;
#2213=CARTESIAN_POINT ( 'NONE',  ( -83.90000000000000568, -35.27268749875867826, 102.5980762113533018 ) ) ;
#2215=CARTESIAN_POINT ( 'NONE',  ( -79.64356964375001269, -35.01562499938548711, 101.5914258081833879 ) ) ;
#2226=CARTESIAN_POINT ( 'NONE',  ( -82.39999999999999147, -32.50312499938548427, 96.81714838363319586 ) ) ;
#2229=EDGE_CURVE ( 'NONE', #4020, #14453, #5179, .T. ) ;
#2232=ORIENTED_EDGE ( 'NONE', *, *, #8150, .T. ) ;
#2237=CARTESIAN_POINT ( 'NONE',  ( -82.39999999999999147, -33.20624999877097139, 96.53589838486223584 ) ) ;
#2238=CARTESIAN_POINT ( 'NONE',  ( -80.90000000000000568, -34.29374999877096997, 102.5980762113533018 ) ) ;
#2255=CARTESIAN_POINT ( 'NONE',  ( -79.39999999999999147, -33.73124999877096997, 98.26794919243110371 ) ) ;
#2261=CARTESIAN_POINT ( 'NONE',  ( -79.39999999999999147, -34.75856250001229597, 101.7320508075688537 ) ) ;
#2269=( BOUNDED_CURVE ( )  B_SPLINE_CURVE ( 2, ( #115, #7422, #13382, #16414, #1663, #16, #4494 ),
 .UNSPECIFIED., .F., .F. ) 
 B_SPLINE_CURVE_WITH_KNOTS ( ( 3, 2, 2, 3 ),
 ( 0.8958333333333333703, 0.9027777777777777901, 0.9166666666666666297, 0.9258785066912882389 ),
 .UNSPECIFIED. ) 
 CURVE ( )  GEOMETRIC_REPRESENTATION_ITEM ( )  RATIONAL_B_SPLINE_CURVE ( ( 0.9330127018922192983, 0.9330127018922198534, 1.000000000000000000, 0.8660254037844387076, 1.000000000000000000, 0.9111410165655264848, 0.9401539157124900736 ) ) 
 REPRESENTATION_ITEM ( '' )  );
#2277=CARTESIAN_POINT ( 'NONE',  ( -81.02178482187500208, -34.90312499938548285, 97.61286128772489690 ) ) ;
#2279=EDGE_LOOP ( 'NONE', ( #4183, #10015, #9450, #7227 ) ) ;
#2286=CARTESIAN_POINT ( 'NONE',  ( -83.77821517812500929, -32.87812499938548427, 102.3871387122750889 ) ) ;
#2294=CARTESIAN_POINT ( 'NONE',  ( -79.39999999999999147, -33.82500000000000284, 99.99999999999998579 ) ) ;
#2302=DIRECTION ( 'NONE',  ( -0.000000000000000000, -1.000000000000000000, -0.000000000000000000 ) ) ;
#2303=CARTESIAN_POINT ( 'NONE',  ( -79.39999999999999147, -30.70856250001229526, 101.7320508075688537 ) ) ;
#2305=CARTESIAN_POINT ( 'NONE',  ( -85.40000000000000568, -33.58518749875867826, 98.26794919243111792 ) ) ;
#2321=CARTESIAN_POINT ( 'NONE',  ( -81.02178482187500208, -33.59062499938548285, 102.3871387122750889 ) ) ;
#2327=VERTEX_POINT ( 'NONE', #11554 ) ;
#2332=CARTESIAN_POINT ( 'NONE',  ( -79.39999999999999147, -33.35624999877097707, 101.7320508075688537 ) ) ;
#2333=CARTESIAN_POINT ( 'NONE',  ( -81.02178482187500208, -31.00312499938548783, 102.3871387122750889 ) ) ;
#2334=CARTESIAN_POINT ( 'NONE',  ( -82.40000000000000568, -30.73124999877097352, 102.9999999999999858 ) ) ;
#2347=CARTESIAN_POINT ( 'NONE',  ( -85.15643035625001289, -30.62812499938548427, 98.40857419181659793 ) ) ;
#2349=CARTESIAN_POINT ( 'NONE',  ( -81.59615242270662350, -32.06115380933863435, 103.0000000000000000 ) ) ;
#2354=EDGE_CURVE ( 'NONE', #15766, #19154, #11162, .T. ) ;
#2357=CARTESIAN_POINT ( 'NONE',  ( -79.39999999999999147, -30.18750000000000355, 98.26794919243110371 ) ) ;
#2361=EDGE_CURVE ( 'NONE', #15766, #19060, #5321, .T. ) ;
#2368=CARTESIAN_POINT ( 'NONE',  ( -82.40000000000001990, -33.20624999877097849, 97.00000000000000000 ) ) ;
#2371=CARTESIAN_POINT ( 'NONE',  ( -79.64356964375001269, -34.56562499938549138, 101.5914258081833879 ) ) ;
#2376=CARTESIAN_POINT ( 'NONE',  ( -82.39999999999999147, -34.52812499938548996, 103.1828516163667899 ) ) ;
#2382=CARTESIAN_POINT ( 'NONE',  ( -85.15643035625001289, -34.26562499938548711, 101.5914258081833879 ) ) ;
#2393=CARTESIAN_POINT ( 'NONE',  ( -80.90000000000000568, -32.40000000000000568, 97.40192378864668399 ) ) ;
#2403=FACE_OUTER_BOUND ( 'NONE', #17857, .T. ) ;
#2404=CARTESIAN_POINT ( 'NONE',  ( -81.02178482187500208, -30.44062499938548783, 102.3871387122750889 ) ) ;
#2419=( GEOMETRIC_REPRESENTATION_CONTEXT ( 3 ) GLOBAL_UNCERTAINTY_ASSIGNED_CONTEXT ( ( #18388 ) ) GLOBAL_UNIT_ASSIGNED_CONTEXT ( ( #5002, #1864, #15640 ) ) REPRESENTATION_CONTEXT ( 'NONE', 'WORKASPACE' ) );
#2432=CARTESIAN_POINT ( 'NONE',  ( -80.90000000000000568, -33.39374999877097139, 102.5980762113533018 ) ) ;
#2433=CARTESIAN_POINT ( 'NONE',  ( -79.64356964375001269, -32.24062499938548854, 98.40857419181659793 ) ) ;
#2436=CIRCLE ( 'NONE', #17096, 7.500000000000020428 ) ;
#2448=CARTESIAN_POINT ( 'NONE',  ( -79.39999999999999147, -35.11874999877096570, 99.99999999999998579 ) ) ;
#2449=CARTESIAN_POINT ( 'NONE',  ( -82.39999999999999147, -30.70312499938548711, 96.81714838363319586 ) ) ;
#2451=ORIENTED_EDGE ( 'NONE', *, *, #12261, .F. ) ;
#2454=CARTESIAN_POINT ( 'NONE',  ( -80.90000000000000568, -33.69374999877096855, 97.40192378864668399 ) ) ;
#2459=CARTESIAN_POINT ( 'NONE',  ( -82.39999999999999147, -34.83356250001229171, 103.4641016151377499 ) ) ;
#2463=CARTESIAN_POINT ( 'NONE',  ( -79.39999999999999147, -33.41250000000000142, 101.7320508075688537 ) ) ;
#2465=CARTESIAN_POINT ( 'NONE',  ( -81.59615242270662350, -31.21740381056766722, 103.0000000000000000 ) ) ;
#2471=CARTESIAN_POINT ( 'NONE',  ( -81.02178482187500208, -33.25312499938548427, 102.3871387122750889 ) ) ;
#2473=ORIENTED_EDGE ( 'NONE', *, *, #6390, .T. ) ;
#2475=CARTESIAN_POINT ( 'NONE',  ( -81.02178482187500208, -34.04062499938548569, 102.3871387122750889 ) ) ;
#2479=CARTESIAN_POINT ( 'NONE',  ( -82.39999999999999147, -34.86562499938548854, 96.81714838363319586 ) ) ;
#2489=CARTESIAN_POINT ( 'NONE',  ( -85.15643035625001289, -30.14062499938548711, 99.99999999999998579 ) ) ;
#2490=CARTESIAN_POINT ( 'NONE',  ( -85.40000000000000568, -32.66250000000000142, 101.7320508075688679 ) ) ;
#2495=FACE_OUTER_BOUND ( 'NONE', #6682, .T. ) ;
#2496=CARTESIAN_POINT ( 'NONE',  ( -79.39999999999999147, -31.08356250001229171, 98.26794919243110371 ) ) ;
#2499=CARTESIAN_POINT ( 'NONE',  ( -81.02178482187500208, -30.74062499938548498, 97.61286128772489690 ) ) ;
#2507=VERTEX_POINT ( 'NONE', #10467 ) ;
#2511=CARTESIAN_POINT ( 'NONE',  ( -81.02178482187500208, -34.94062499938548427, 102.3871387122750889 ) ) ;
#2515=DIRECTION ( 'NONE',  ( -0.000000000000000000, -1.000000000000000000, -0.000000000000000000 ) ) ;
#2521=CARTESIAN_POINT ( 'NONE',  ( -84.69814161231455785, -35.39427329483935836, 98.07164704222793716 ) ) ;
#2522=CARTESIAN_POINT ( 'NONE',  ( -79.64356964374999848, -31.37812499938548427, 99.99999999999998579 ) ) ;
#2532=CARTESIAN_POINT ( 'NONE',  ( -82.39999999999999147, -30.92812499938548143, 103.1828516163667899 ) ) ;
#2543=CARTESIAN_POINT ( 'NONE',  ( -80.90000000000000568, -32.10000000000000142, 102.5980762113533018 ) ) ;
#2550=VERTEX_POINT ( 'NONE', #10284 ) ;
#2553=VECTOR ( 'NONE', #2515, 1000.000000000000000 ) ;
#2557=CARTESIAN_POINT ( 'NONE',  ( -83.77821517812500929, -32.87812499938548427, 102.3871387122750889 ) ) ;
#2562=CARTESIAN_POINT ( 'NONE',  ( -81.02178482187500208, -33.89062499938548711, 97.61286128772489690 ) ) ;
#2563=EDGE_CURVE ( 'NONE', #11976, #6642, #13389, .T. ) ;
#2571=CARTESIAN_POINT ( 'NONE',  ( -79.64356964374998427, -33.59062499938548285, 98.40857419181659793 ) ) ;
#2580=CYLINDRICAL_SURFACE ( 'NONE', #8809, 3.000000000000002665 ) ;
#2582=CARTESIAN_POINT ( 'NONE',  ( -82.39999999999999147, -32.81250000000000000, 96.53589838486223584 ) ) ;
#2586=DIRECTION ( 'NONE',  ( -0.000000000000000000, -1.000000000000000000, -0.000000000000000000 ) ) ;
#2593=CARTESIAN_POINT ( 'NONE',  ( -83.77821517812500929, -30.21562499938548285, 97.61286128772489690 ) ) ;
#2600=ORIENTED_EDGE ( 'NONE', *, *, #13152, .F. ) ;
#2605=( BOUNDED_CURVE ( )  B_SPLINE_CURVE ( 1, ( #1455, #6243 ),
 .UNSPECIFIED., .F., .F. ) 
 B_SPLINE_CURVE_WITH_KNOTS ( ( 2, 2 ),
 ( 0.000000000000000000, 1.000000000000000000 ),
 .UNSPECIFIED. ) 
 CURVE ( )  GEOMETRIC_REPRESENTATION_ITEM ( )  RATIONAL_B_SPLINE_CURVE ( ( 0.9401542295229963209, 0.9401542295229963209 ) ) 
 REPRESENTATION_ITEM ( '' )  );
#2616=CARTESIAN_POINT ( 'NONE',  ( -82.39999999999999147, -30.51018749875868252, 96.53589838486223584 ) ) ;
#2617=CARTESIAN_POINT ( 'NONE',  ( -79.64356964375001269, -31.79062499938548569, 98.40857419181659793 ) ) ;
#2627=CARTESIAN_POINT ( 'NONE',  ( -82.39999999999999147, -31.82812499938548356, 103.1828516163667899 ) ) ;
#2638=CARTESIAN_POINT ( 'NONE',  ( -79.39999999999999147, -31.08750000000000213, 98.26794919243110371 ) ) ;
#2649=AXIS2_PLACEMENT_3D ( 'NONE', #7712, #1755, #9366 ) ;
#2653=CARTESIAN_POINT ( 'NONE',  ( -79.64356964374999848, -30.81562499938548427, 99.99999999999998579 ) ) ;
#2659=CARTESIAN_POINT ( 'NONE',  ( -82.39999999999999147, -33.40312499938548285, 96.81714838363319586 ) ) ;
#2671=EDGE_CURVE ( 'NONE', #19154, #12568, #4037, .T. ) ;
#2679=CARTESIAN_POINT ( 'NONE',  ( -83.90000000000000568, -32.62500000000000000, 102.5980762113533018 ) ) ;
#2687=CARTESIAN_POINT ( 'NONE',  ( -82.39999999999999147, -30.10856250001229384, 96.53589838486223584 ) ) ;
#2689=CARTESIAN_POINT ( 'NONE',  ( -82.39999999999999147, -34.83749999999999858, 103.0000000000000000 ) ) ;
#2692=CARTESIAN_POINT ( 'NONE',  ( -83.90000000000000568, -32.56874999877096855, 102.5980762113533018 ) ) ;
#2707=ORIENTED_EDGE ( 'NONE', *, *, #8266, .T. ) ;
#2713=ADVANCED_FACE ( 'NONE', ( #15547 ), #15346, .T. ) ;
#2717=CARTESIAN_POINT ( 'NONE',  ( -83.90000000000000568, -30.47268749875867755, 97.40192378864668399 ) ) ;
#2719=CARTESIAN_POINT ( 'NONE',  ( -81.02178482187500208, -31.30312499938548498, 97.61286128772489690 ) ) ;
#2731=CARTESIAN_POINT ( 'NONE',  ( -81.02178482187500208, -30.29062499938548569, 97.61286128772489690 ) ) ;
#2739=CARTESIAN_POINT ( 'NONE',  ( -82.39999999999999147, -31.85624999877096641, 96.99999999999998579 ) ) ;
#2744=CARTESIAN_POINT ( 'NONE',  ( -79.39999999999999147, -32.92500000000000426, 99.99999999999998579 ) ) ;
#2757=CARTESIAN_POINT ( 'NONE',  ( -79.39999999999999147, -33.28124999877096712, 98.26794919243110371 ) ) ;
#2759=CARTESIAN_POINT ( 'NONE',  ( -83.77821517812500929, -31.56562499938548427, 97.61286128772489690 ) ) ;
#2765=CARTESIAN_POINT ( 'NONE',  ( -85.15643035624999868, -33.25312499938548427, 101.5914258081833879 ) ) ;
#2781=DIRECTION ( 'NONE',  ( -0.000000000000000000, -1.000000000000000000, -0.000000000000000000 ) ) ;
#2784=( BOUNDED_CURVE ( )  B_SPLINE_CURVE ( 2, ( #7473, #16463, #11676, #7184, #11581, #4255, #17544, #10214, #2787 ),
 .UNSPECIFIED., .F., .F. ) 
 B_SPLINE_CURVE_WITH_KNOTS ( ( 3, 2, 2, 2, 3 ),
 ( 0.06250000000000002776, 0.06944444444444444753, 0.08333333333333332871, 0.09722222222222222376, 0.1041666666666666713 ),
 .UNSPECIFIED. ) 
 CURVE ( )  GEOMETRIC_REPRESENTATION_ITEM ( )  RATIONAL_B_SPLINE_CURVE ( ( 0.9330127018922194093, 0.9330127018922196314, 1.000000000000000000, 0.8660254037844387076, 1.000000000000000000, 0.8660254037844387076, 1.000000000000000000, 0.9330127018922192983, 0.9330127018922194093 ) ) 
 REPRESENTATION_ITEM ( '' )  );
#2787=CARTESIAN_POINT ( 'NONE',  ( -82.40000000000000568, -30.56250000000001066, 96.99999999999998579 ) ) ;
#2789=ADVANCED_FACE ( 'NONE', ( #9287 ), #15444, .T. ) ;
#2792=CARTESIAN_POINT ( 'NONE',  ( -83.90000000000000568, -31.72106250001229810, 102.5980762113533018 ) ) ;
#2795=CARTESIAN_POINT ( 'NONE',  ( -79.64356964374999848, -30.81562499938548427, 99.99999999999998579 ) ) ;
#2812=VERTEX_POINT ( 'NONE', #4814 ) ;
#2818=CARTESIAN_POINT ( 'NONE',  ( -83.90000000000000568, -33.46874999877096712, 102.5980762113533018 ) ) ;
#2819=CARTESIAN_POINT ( 'NONE',  ( -85.15643035624999868, -34.34062499938548285, 98.40857419181659793 ) ) ;
#2831=CARTESIAN_POINT ( 'NONE',  ( -85.15643035625001289, -34.22812499938548569, 98.40857419181659793 ) ) ;
#2841=CARTESIAN_POINT ( 'NONE',  ( -85.40000000000000568, -31.83750000000000568, 98.26794919243111792 ) ) ;
#2846=CARTESIAN_POINT ( 'NONE',  ( -84.69814099439363986, -35.09873396208577390, 98.07164630581206666 ) ) ;
#2852=CYLINDRICAL_SURFACE ( 'NONE', #16778, 3.000000000000002665 ) ;
#2855=CARTESIAN_POINT ( 'NONE',  ( -81.02178482187500208, -35.05312499938548854, 102.3871387122750889 ) ) ;
#2861=CARTESIAN_POINT ( 'NONE',  ( -80.90000000000000568, -32.10000000000000142, 102.5980762113533018 ) ) ;
#2868=AXIS2_PLACEMENT_3D ( 'NONE', #18269, #13954, #9665 ) ;
#2876=DIRECTION ( 'NONE',  ( -0.000000000000000000, -1.000000000000000000, -0.000000000000000000 ) ) ;
#2885=CARTESIAN_POINT ( 'NONE',  ( -82.39999999999999147, -32.58356250001229881, 103.4641016151377499 ) ) ;
#2888=CARTESIAN_POINT ( 'NONE',  ( -83.77821517812500929, -30.96562499938548640, 102.3871387122750889 ) ) ;
#2907=CARTESIAN_POINT ( 'NONE',  ( -79.39999999999999147, -30.26250000000000284, 101.7320508075688537 ) ) ;
#2913=CARTESIAN_POINT ( 'NONE',  ( -85.40000000000000568, -32.61018749875868394, 101.7320508075688679 ) ) ;
#2914=CARTESIAN_POINT ( 'NONE',  ( -79.64356964375001269, -32.76562499938548711, 101.5914258081833879 ) ) ;
#2921=ORIENTED_EDGE ( 'NONE', *, *, #8685, .T. ) ;
#2926=CARTESIAN_POINT ( 'NONE',  ( -79.64356964374999848, -33.96562499938548285, 99.99999999999998579 ) ) ;
#2936=CARTESIAN_POINT ( 'NONE',  ( -82.39999999999999147, -33.71249999999999858, 96.53589838486223584 ) ) ;
#2937=EDGE_CURVE ( 'NONE', #3433, #6642, #16534, .T. ) ;
#2938=CARTESIAN_POINT ( 'NONE',  ( -80.90000000000000568, -30.99374999877096926, 97.40192378864668399 ) ) ;
#2939=CARTESIAN_POINT ( 'NONE',  ( -82.40000000000000568, -30.00000000000000355, 99.99999999999998579 ) ) ;
#2946=CARTESIAN_POINT ( 'NONE',  ( -84.51155386534844638, -35.25364837475780888, 98.22820752270799005 ) ) ;
#2948=CARTESIAN_POINT ( 'NONE',  ( -79.64356964374999848, -32.16562499938548569, 99.99999999999998579 ) ) ;
#2950=EDGE_CURVE ( 'NONE', #3433, #6725, #4244, .T. ) ;
#2955=CARTESIAN_POINT ( 'NONE',  ( -83.90000000000000568, -30.97500000000000142, 97.40192378864668399 ) ) ;
#2970=CARTESIAN_POINT ( 'NONE',  ( -85.40000000000000568, -34.93124999877096570, 98.26794919243111792 ) ) ;
#2977=CARTESIAN_POINT ( 'NONE',  ( -79.39999999999999147, -32.47106250001229455, 99.99999999999998579 ) ) ;
#2980=CARTESIAN_POINT ( 'NONE',  ( -83.77821517812500929, -32.46562499938548285, 97.61286128772489690 ) ) ;
#3004=CARTESIAN_POINT ( 'NONE',  ( -83.90000000000000568, -31.67268749875867684, 102.5980762113533018 ) ) ;
#3005=CARTESIAN_POINT ( 'NONE',  ( -85.15643035624999868, -32.54062499938548569, 98.40857419181659793 ) ) ;
#3006=CARTESIAN_POINT ( 'NONE',  ( -79.39999999999999147, -31.57499999999999929, 99.99999999999998579 ) ) ;
#3013=ADVANCED_FACE ( 'NONE', ( #16671 ), #11981, .T. ) ;
#3018=CARTESIAN_POINT ( 'NONE',  ( -81.02178482187500208, -33.14062499938548711, 102.3871387122750889 ) ) ;
#3024=ORIENTED_EDGE ( 'NONE', *, *, #18429, .T. ) ;
#3028=EDGE_CURVE ( 'NONE', #14891, #19060, #15384, .T. ) ;
#3030=CARTESIAN_POINT ( 'NONE',  ( -79.39999999999999147, -34.72500000000000142, 99.99999999999998579 ) ) ;
#3032=CARTESIAN_POINT ( 'NONE',  ( -79.39999999999999147, -31.03124999877097068, 98.26794919243110371 ) ) ;
#3044=CARTESIAN_POINT ( 'NONE',  ( -79.64356964374999848, -31.71562499938548285, 99.99999999999998579 ) ) ;
#3051=CARTESIAN_POINT ( 'NONE',  ( -82.39999999999999147, -31.91250000000000497, 96.53589838486223584 ) ) ;
#3058=CARTESIAN_POINT ( 'NONE',  ( -82.40000000000001990, -33.88124999877096855, 103.0000000000000000 ) ) ;
#3067=CARTESIAN_POINT ( 'NONE',  ( -79.39999999999999147, -34.72500000000000142, 99.99999999999998579 ) ) ;
#3073=CARTESIAN_POINT ( 'NONE',  ( -82.40000000000000568, -34.10624999877096997, 96.99999999999998579 ) ) ;
#3074=CARTESIAN_POINT ( 'NONE',  ( -85.40000000000000568, -31.34606250001229810, 99.99999999999998579 ) ) ;
#3077=CARTESIAN_POINT ( 'NONE',  ( -85.15643035624999868, -31.45312499938548356, 101.5914258081833879 ) ) ;
#3098=CARTESIAN_POINT ( 'NONE',  ( -80.90000000000000568, -32.94768749875867542, 102.5980762113533018 ) ) ;
#3100=CARTESIAN_POINT ( 'NONE',  ( -85.15643035624999868, -34.79062499938548569, 98.40857419181659793 ) ) ;
#3105=CARTESIAN_POINT ( 'NONE',  ( -82.40000000000000568, -30.00000000000000355, 103.0000000000000000 ) ) ;
#3112=CARTESIAN_POINT ( 'NONE',  ( -79.64356964374999848, -32.61562499938548854, 99.99999999999998579 ) ) ;
#3114=ORIENTED_EDGE ( 'NONE', *, *, #18600, .F. ) ;
#3118=ORIENTED_EDGE ( 'NONE', *, *, #5910, .T. ) ;
#3119=CARTESIAN_POINT ( 'NONE',  ( -82.40000000000000568, -50.00000000000000000, 92.49999999999997158 ) ) ;
#3123=CARTESIAN_POINT ( 'NONE',  ( -80.90000000000000568, -30.54374999877096997, 97.40192378864668399 ) ) ;
#3124=CARTESIAN_POINT ( 'NONE',  ( -85.40000000000000568, -30.84374999877096712, 99.99999999999998579 ) ) ;
#3131=SURFACE_STYLE_USAGE ( .BOTH. , #18189 ) ;
#3136=CARTESIAN_POINT ( 'NONE',  ( -79.64356964375001269, -33.47812499938547859, 98.40857419181659793 ) ) ;
#3142=CARTESIAN_POINT ( 'NONE',  ( -83.90000000000000568, -30.52500000000000213, 97.40192378864668399 ) ) ;
#3163=CARTESIAN_POINT ( 'NONE',  ( -83.18600968418431307, -35.00069049296057955, 102.9003918199492915 ) ) ;
#3168=CARTESIAN_POINT ( 'NONE',  ( -82.39999999999999147, -31.90856250001229810, 96.53589838486223584 ) ) ;
#3175=FACE_OUTER_BOUND ( 'NONE', #9076, .T. ) ;
#3179=DIRECTION ( 'NONE',  ( 0.000000000000000000, 0.000000000000000000, -1.000000000000000000 ) ) ;
#3181=CARTESIAN_POINT ( 'NONE',  ( -83.20384757729335945, -33.05759618943233136, 102.9999999999999858 ) ) ;
#3186=EDGE_CURVE ( 'NONE', #12568, #1155, #11648, .T. ) ;
#3193=CARTESIAN_POINT ( 'NONE',  ( -79.39999999999999147, -30.66018749875867755, 101.7320508075688537 ) ) ;
#3195=CARTESIAN_POINT ( 'NONE',  ( -85.15643035624999868, -33.89062499938548711, 98.40857419181659793 ) ) ;
#3209=CARTESIAN_POINT ( 'NONE',  ( -79.64356964374998427, -34.00312499938548427, 101.5914258081833879 ) ) ;
#3216=ORIENTED_EDGE ( 'NONE', *, *, #2563, .T. ) ;
#3217=CARTESIAN_POINT ( 'NONE',  ( -83.90000000000000568, -31.36874999877096926, 97.40192378864668399 ) ) ;
#3220=CARTESIAN_POINT ( 'NONE',  ( -82.39999999999999147, -34.16250000000000142, 96.53589838486223584 ) ) ;
#3221=CARTESIAN_POINT ( 'NONE',  ( -85.40000000000000568, -31.25624999877096855, 101.7320508075688679 ) ) ;
#3222=FACE_OUTER_BOUND ( 'NONE', #204, .T. ) ;
#3239=CARTESIAN_POINT ( 'NONE',  ( -85.40000000000000568, -31.83750000000000568, 98.26794919243111792 ) ) ;
#3247=ORIENTED_EDGE ( 'NONE', *, *, #17486, .T. ) ;
#3254=CARTESIAN_POINT ( 'NONE',  ( -85.15643035624999868, -32.09062499938548996, 98.40857419181659793 ) ) ;
#3258=CARTESIAN_POINT ( 'NONE',  ( -79.43507259642450435, -35.00111651776678201, 99.51279508880003277 ) ) ;
#3260=CARTESIAN_POINT ( 'NONE',  ( -80.90000000000000568, -32.55000000000000426, 102.5980762113533018 ) ) ;
#3261=CARTESIAN_POINT ( 'NONE',  ( -82.39999999999999147, -34.38356250001228176, 103.4641016151377499 ) ) ;
#3265=CARTESIAN_POINT ( 'NONE',  ( -79.64356964374998427, -31.86562499938548143, 101.5914258081833879 ) ) ;
#3280=FACE_OUTER_BOUND ( 'NONE', #14173, .T. ) ;
#3288=CARTESIAN_POINT ( 'NONE',  ( -85.40000000000000568, -31.26018749875867186, 101.7320508075688679 ) ) ;
#3289=CARTESIAN_POINT ( 'NONE',  ( -84.51155386534844638, -35.25364837475780888, 98.22820752270799005 ) ) ;
#3296=ADVANCED_FACE ( 'NONE', ( #10089 ), #14377, .T. ) ;
#3304=CARTESIAN_POINT ( 'NONE',  ( -83.77821517812500929, -35.01562499938548711, 102.3871387122750889 ) ) ;
#3309=AXIS2_PLACEMENT_3D ( 'NONE', #14269, #718, #13985 ) ;
#3314=CARTESIAN_POINT ( 'NONE',  ( -80.90000000000000568, -33.75000000000000000, 97.40192378864668399 ) ) ;
#3315=CARTESIAN_POINT ( 'NONE',  ( -83.90000000000000568, -34.12500000000000000, 97.40192378864668399 ) ) ;
#3317=CARTESIAN_POINT ( 'NONE',  ( -80.90000000000000568, -33.39374999877097139, 102.5980762113533018 ) ) ;
#3331=CARTESIAN_POINT ( 'NONE',  ( -80.90000000000000568, -30.15000000000000213, 97.40192378864668399 ) ) ;
#3345=ADVANCED_FACE ( 'NONE', ( #17903 ), #2852, .T. ) ;
#3355=CARTESIAN_POINT ( 'NONE',  ( -79.64356964375001269, -30.51562499938548711, 101.5914258081833879 ) ) ;
#3358=ORIENTED_EDGE ( 'NONE', *, *, #4450, .T. ) ;
#3368=CARTESIAN_POINT ( 'NONE',  ( -79.64356964374998427, -30.89062499938548711, 98.40857419181659793 ) ) ;
#3392=CARTESIAN_POINT ( 'NONE',  ( -85.40000000000000568, -33.09768749875867400, 99.99999999999998579 ) ) ;
#3406=CARTESIAN_POINT ( 'NONE',  ( -81.02178482187500208, -34.94062499938548427, 102.3871387122750889 ) ) ;
#3408=EDGE_LOOP ( 'NONE', ( #5079, #441, #8494, #13671 ) ) ;
#3410=( BOUNDED_CURVE ( )  B_SPLINE_CURVE ( 2, ( #1524, #11866, #17834, #61, #18224, #6015, #1798, #9126, #11961 ),
 .UNSPECIFIED., .F., .F. ) 
 B_SPLINE_CURVE_WITH_KNOTS ( ( 3, 2, 2, 2, 3 ),
 ( 0.1041666666666666713, 0.1111111111111111049, 0.1250000000000000000, 0.1388888888888888951, 0.1458333333333334814 ),
 .UNSPECIFIED. ) 
 CURVE ( )  GEOMETRIC_REPRESENTATION_ITEM ( )  RATIONAL_B_SPLINE_CURVE ( ( 0.9330127018922194093, 0.9330127018922194093, 1.000000000000000000, 0.8660254037844387076, 1.000000000000000000, 0.8660254037844387076, 1.000000000000000000, 0.9330127018922180770, 0.9330127018922194093 ) ) 
 REPRESENTATION_ITEM ( '' )  );
#3416=CARTESIAN_POINT ( 'NONE',  ( -82.39999999999999147, -34.16250000000000142, 97.00000000000000000 ) ) ;
#3417=CARTESIAN_POINT ( 'NONE',  ( -80.90000000000000568, -31.59374999877097423, 102.5980762113533018 ) ) ;
#3418=CARTESIAN_POINT ( 'NONE',  ( -82.39999999999999147, -33.43124999877097281, 103.4641016151377499 ) ) ;
#3433=VERTEX_POINT ( 'NONE', #132 ) ;
#3437=( BOUNDED_CURVE ( )  B_SPLINE_CURVE ( 2, ( #11845, #17813, #10190, #7256, #10577, #17720, #8907, #12037, #4623 ),
 .UNSPECIFIED., .F., .F. ) 
 B_SPLINE_CURVE_WITH_KNOTS ( ( 3, 2, 2, 2, 3 ),
 ( 0.3125000000000001110, 0.3194444444444444198, 0.3333333333333333148, 0.3472222222222222099, 0.3541666666666666852 ),
 .UNSPECIFIED. ) 
 CURVE ( )  GEOMETRIC_REPRESENTATION_ITEM ( )  RATIONAL_B_SPLINE_CURVE ( ( 0.9330127018922194093, 0.9330127018922204085, 1.000000000000000000, 0.8660254037844387076, 1.000000000000000000, 0.8660254037844387076, 1.000000000000000000, 0.9330127018922190762, 0.9330127018922194093 ) ) 
 REPRESENTATION_ITEM ( '' )  );
#3442=CARTESIAN_POINT ( 'NONE',  ( -82.40000000000000568, -30.00000000000000355, 103.0000000000000000 ) ) ;
#3451=CARTESIAN_POINT ( 'NONE',  ( -83.77821517812500929, -32.57812499938548711, 97.61286128772489690 ) ) ;
#3459=CARTESIAN_POINT ( 'NONE',  ( -79.64356964374998427, -30.96562499938548640, 101.5914258081833879 ) ) ;
#3480=CARTESIAN_POINT ( 'NONE',  ( -83.90000000000000568, -33.17268749875866973, 97.40192378864668399 ) ) ;
#3483=CARTESIAN_POINT ( 'NONE',  ( -85.40000000000000568, -34.44374999877096855, 99.99999999999998579 ) ) ;
#3497=CARTESIAN_POINT ( 'NONE',  ( -85.15643035625001289, -32.39062499938548711, 99.99999999999998579 ) ) ;
#3499=ORIENTED_EDGE ( 'NONE', *, *, #9854, .T. ) ;
#3502=CARTESIAN_POINT ( 'NONE',  ( -83.90000000000000568, -30.91874999877096997, 97.40192378864668399 ) ) ;
#3510=CARTESIAN_POINT ( 'NONE',  ( -85.40000000000000568, -31.25624999877096855, 101.7320508075688679 ) ) ;
#3511=CARTESIAN_POINT ( 'NONE',  ( -80.90000000000000568, -33.84374999877096712, 102.5980762113533018 ) ) ;
#3523=( BOUNDED_CURVE ( )  B_SPLINE_CURVE ( 2, ( #4770, #3768, #9436, #3576, #8363, #10905, #9735, #5147, #9642 ),
 .UNSPECIFIED., .F., .F. ) 
 B_SPLINE_CURVE_WITH_KNOTS ( ( 3, 2, 2, 2, 3 ),
 ( 0.3541666666666666297, 0.3611111111111111049, 0.3750000000000000000, 0.3888888888888888951, 0.3958333333333334259 ),
 .UNSPECIFIED. ) 
 CURVE ( )  GEOMETRIC_REPRESENTATION_ITEM ( )  RATIONAL_B_SPLINE_CURVE ( ( 0.9330127018922194093, 0.9330127018922190762, 1.000000000000000000, 0.8660254037844387076, 1.000000000000000000, 0.8660254037844387076, 1.000000000000000000, 0.9330127018922185211, 0.9330127018922192983 ) ) 
 REPRESENTATION_ITEM ( '' )  );
#3526=CLOSED_SHELL ( 'NONE', ( #5779, #17132, #6134, #11799, #1815, #10200, #17470, #1365, #19082, #4921, #3013, #6402, #15074, #16330, #934, #7816, #3296, #10940, #3345, #18227, #18400, #9723, #17020, #2713, #650, #905, #12213, #2789, #10924, #11662, #667, #8417, #17025, #13751 ) ) ;
#3542=CARTESIAN_POINT ( 'NONE',  ( -80.90000000000000568, -33.30000000000000426, 97.40192378864668399 ) ) ;
#3545=ORIENTED_EDGE ( 'NONE', *, *, #8064, .T. ) ;
#3549=CARTESIAN_POINT ( 'NONE',  ( -85.40000000000000568, -34.03124999877096712, 98.26794919243111792 ) ) ;
#3551=CARTESIAN_POINT ( 'NONE',  ( -79.64356964374999848, -31.37812499938548427, 99.99999999999998579 ) ) ;
#3554=EDGE_LOOP ( 'NONE', ( #6738, #7388, #9688, #4859 ) ) ;
#3560=CARTESIAN_POINT ( 'NONE',  ( -85.15643035625001289, -31.56562499938548427, 101.5914258081833879 ) ) ;
#3576=CARTESIAN_POINT ( 'NONE',  ( -79.39999999999999147, -32.38124999877096855, 98.26794919243110371 ) ) ;
#3579=CARTESIAN_POINT ( 'NONE',  ( -79.39999999999999147, -35.08518749875868536, 98.26794919243110371 ) ) ;
#3582=CARTESIAN_POINT ( 'NONE',  ( -81.02178482187500208, -35.05312499938548854, 102.3871387122750889 ) ) ;
#3583=CARTESIAN_POINT ( 'NONE',  ( -85.40000000000000568, -34.48124999877096997, 98.26794919243111792 ) ) ;
#3594=CARTESIAN_POINT ( 'NONE',  ( -81.02178482187500208, -34.34062499938548285, 97.61286128772489690 ) ) ;
#3604=LINE ( 'NONE', #12308, #12554 ) ;
#3605=CARTESIAN_POINT ( 'NONE',  ( -82.39999999999999147, -32.75624999877096855, 96.53589838486223584 ) ) ;
#3606=CARTESIAN_POINT ( 'NONE',  ( -82.39999999999999147, -32.98124999877096997, 103.4641016151377499 ) ) ;
#3607=CARTESIAN_POINT ( 'NONE',  ( -83.90000000000000568, -32.32500000000000284, 97.40192378864668399 ) ) ;
#3608=EDGE_CURVE ( 'NONE', #10334, #4020, #706, .T. ) ;
#3613=EDGE_LOOP ( 'NONE', ( #2473, #9269, #13788, #9361 ) ) ;
#3622=ORIENTED_EDGE ( 'NONE', *, *, #10828, .T. ) ;
#3632=CARTESIAN_POINT ( 'NONE',  ( -80.90000000000000568, -33.89606250001229171, 102.5980762113533018 ) ) ;
#3647=CARTESIAN_POINT ( 'NONE',  ( -81.02178482187500208, -31.30312499938548498, 97.61286128772489690 ) ) ;
#3657=CARTESIAN_POINT ( 'NONE',  ( -85.15643035625001289, -32.95312499938548711, 99.99999999999998579 ) ) ;
#3672=CARTESIAN_POINT ( 'NONE',  ( -85.40000000000000568, -31.31250000000000000, 101.7320508075688821 ) ) ;
#3677=DIRECTION ( 'NONE',  ( 0.000000000000000000, 0.000000000000000000, -1.000000000000000000 ) ) ;
#3679=CARTESIAN_POINT ( 'NONE',  ( -81.59615242270665192, -32.77634618820330559, 97.00000000000000000 ) ) ;
#3681=CARTESIAN_POINT ( 'NONE',  ( -80.90000000000000568, -33.69768749875867542, 97.40192378864668399 ) ) ;
#3686=CARTESIAN_POINT ( 'NONE',  ( -82.40000000000000568, -30.00000000000000355, 99.99999999999998579 ) ) ;
#3694=CARTESIAN_POINT ( 'NONE',  ( -85.15643035624999868, -33.32812499938548001, 98.40857419181659793 ) ) ;
#3696=ORIENTED_EDGE ( 'NONE', *, *, #7022, .F. ) ;
#3704=CARTESIAN_POINT ( 'NONE',  ( -80.90000000000000568, -34.35000000000000853, 102.5980762113533018 ) ) ;
#3705=CARTESIAN_POINT ( 'NONE',  ( -79.39999999999999147, -32.41874999877096997, 99.99999999999998579 ) ) ;
#3706=CARTESIAN_POINT ( 'NONE',  ( -85.40000000000000568, -34.48124999877096997, 98.26794919243111792 ) ) ;
#3717=DIRECTION ( 'NONE',  ( 0.000000000000000000, 1.000000000000000000, 0.000000000000000000 ) ) ;
#3726=CARTESIAN_POINT ( 'NONE',  ( -83.90000000000000568, -30.46874999877096712, 97.40192378864668399 ) ) ;
#3728=CARTESIAN_POINT ( 'NONE',  ( -82.39999999999999147, -30.56250000000000355, 96.53589838486223584 ) ) ;
#3734=CARTESIAN_POINT ( 'NONE',  ( -82.39999999999999147, -31.01249999999999929, 96.99999999999998579 ) ) ;
#3740=CARTESIAN_POINT ( 'NONE',  ( -79.64356964375001269, -33.14062499938548711, 98.40857419181659793 ) ) ;
#3743=EDGE_LOOP ( 'NONE', ( #11940, #1148, #11091, #1297 ) ) ;
#3750=CARTESIAN_POINT ( 'NONE',  ( -83.77821517812500929, -34.82812499938548711, 97.61286128772489690 ) ) ;
#3762=CARTESIAN_POINT ( 'NONE',  ( -85.40000000000000568, -33.63750000000000284, 98.26794919243111792 ) ) ;
#3768=CARTESIAN_POINT ( 'NONE',  ( -81.59615242270660929, -32.32634618820329564, 96.99999999999997158 ) ) ;
#3770=CARTESIAN_POINT ( 'NONE',  ( -79.39999999999999147, -30.63356250001229242, 98.26794919243110371 ) ) ;
#3771=CARTESIAN_POINT ( 'NONE',  ( -82.39999999999999147, -34.11018749875866973, 96.53589838486223584 ) ) ;
#3786=CARTESIAN_POINT ( 'NONE',  ( -85.15643035625001289, -34.19062499938548427, 99.99999999999998579 ) ) ;
#3790=CARTESIAN_POINT ( 'NONE',  ( -85.15643035625001289, -30.14062499938548711, 99.99999999999998579 ) ) ;
#3796=CARTESIAN_POINT ( 'NONE',  ( -82.39999999999999147, -32.53124999877096712, 103.4641016151377499 ) ) ;
#3797=CARTESIAN_POINT ( 'NONE',  ( -85.15643035625001289, -30.70312499938548711, 99.99999999999998579 ) ) ;
#3809=CARTESIAN_POINT ( 'NONE',  ( -81.02178482187500208, -30.44062499938548783, 102.3871387122750889 ) ) ;
#3820=CARTESIAN_POINT ( 'NONE',  ( -85.40000000000000568, -29.97835047384105067, 100.9999487804559664 ) ) ;
#3831=DIRECTION ( 'NONE',  ( -0.000000000000000000, -1.000000000000000000, -0.000000000000000000 ) ) ;
#3834=CARTESIAN_POINT ( 'NONE',  ( -82.39999999999999147, -33.29062499938549280, 103.1828516163667899 ) ) ;
#3838=CARTESIAN_POINT ( 'NONE',  ( -80.98256025945210013, -35.00066800082266383, 97.35069876254466692 ) ) ;
#3839=CARTESIAN_POINT ( 'NONE',  ( -85.15643035624999868, -35.05312499938548143, 101.5914258081833879 ) ) ;
#3841=CARTESIAN_POINT ( 'NONE',  ( -84.70833260042415702, -35.00006955123599539, 98.08383195543535749 ) ) ;
#3846=CARTESIAN_POINT ( 'NONE',  ( -85.15643035625001289, -34.34062499938548285, 98.40857419181659793 ) ) ;
#3860=CARTESIAN_POINT ( 'NONE',  ( -82.39999999999999147, -33.26250000000000284, 96.53589838486223584 ) ) ;
#3868=CARTESIAN_POINT ( 'NONE',  ( -82.40000000000000568, -30.00000000000000355, 96.99999999999998579 ) ) ;
#3871=CARTESIAN_POINT ( 'NONE',  ( -81.59615242270662350, -34.63259618943234130, 96.99999999999997158 ) ) ;
#3873=CARTESIAN_POINT ( 'NONE',  ( -79.64356964374999848, -30.36562499938548498, 99.99999999999998579 ) ) ;
#3885=CARTESIAN_POINT ( 'NONE',  ( -83.77821517812500929, -35.01562499938548711, 102.3871387122750889 ) ) ;
#3894=CARTESIAN_POINT ( 'NONE',  ( -83.90000000000000568, -34.51874999877097139, 97.40192378864668399 ) ) ;
#3896=CARTESIAN_POINT ( 'NONE',  ( -85.15643035624999868, -30.74062499938548143, 98.40857419181659793 ) ) ;
#3909=CARTESIAN_POINT ( 'NONE',  ( -85.15643035625001289, -31.45312499938548356, 101.5914258081833879 ) ) ;
#3910=DIRECTION ( 'NONE',  ( 0.000000000000000000, -1.000000000000000000, 0.000000000000000000 ) ) ;
#3914=LINE ( 'NONE', #8313, #5382 ) ;
#3921=CARTESIAN_POINT ( 'NONE',  ( -83.90000000000000568, -30.82500000000000284, 102.5980762113533018 ) ) ;
#3929=CARTESIAN_POINT ( 'NONE',  ( -79.39999999999999147, -31.16249999999999787, 101.7320508075688537 ) ) ;
#3935=CARTESIAN_POINT ( 'NONE',  ( -81.02178482187500208, -34.60312499938549280, 102.3871387122750889 ) ) ;
#3939=CARTESIAN_POINT ( 'NONE',  ( -82.39999999999999147, -33.62812499938549138, 103.1828516163667899 ) ) ;
#3947=CARTESIAN_POINT ( 'NONE',  ( -79.64356964374998427, -34.49062499938548854, 98.40857419181659793 ) ) ;
#3955=ORIENTED_EDGE ( 'NONE', *, *, #7675, .T. ) ;
#3958=CARTESIAN_POINT ( 'NONE',  ( -82.39999999999999147, -34.61250000000000426, 96.53589838486223584 ) ) ;
#3964=CARTESIAN_POINT ( 'NONE',  ( -82.40000000000000568, -30.11250000000000071, 96.99999999999998579 ) ) ;
#3965=CARTESIAN_POINT ( 'NONE',  ( -85.40000000000000568, -29.99606250001229313, 99.99999999999998579 ) ) ;
#3969=CARTESIAN_POINT ( 'NONE',  ( -85.15643035624999868, -30.62812499938548427, 98.40857419181659793 ) ) ;
#3997=CARTESIAN_POINT ( 'NONE',  ( -85.40000000000000568, -33.50624999877096855, 101.7320508075688679 ) ) ;
#3998=CARTESIAN_POINT ( 'NONE',  ( -83.77821517812500929, -30.32812499938548711, 97.61286128772489690 ) ) ;
#4001=VECTOR ( 'NONE', #7169, 1000.000000000000000 ) ;
#4013=CARTESIAN_POINT ( 'NONE',  ( -84.44489485864974654, -35.00000000000000000, 97.76983701218843237 ) ) ;
#4014=CARTESIAN_POINT ( 'NONE',  ( -79.64356964374998427, -30.32812499938548711, 98.40857419181659793 ) ) ;
#4017=CARTESIAN_POINT ( 'NONE',  ( -82.40000000000000568, -32.08124999877097139, 102.9999999999999858 ) ) ;
#4020=VERTEX_POINT ( 'NONE', #1395 ) ;
#4025=CARTESIAN_POINT ( 'NONE',  ( -80.90000000000000568, -33.30000000000000426, 97.40192378864668399 ) ) ;
#4037=( BOUNDED_CURVE ( )  B_SPLINE_CURVE ( 2, ( #16720, #2057, #613, #6562, #5100, #18579, #8014, #13689, #5007 ),
 .UNSPECIFIED., .F., .F. ) 
 B_SPLINE_CURVE_WITH_KNOTS ( ( 3, 2, 2, 2, 3 ),
 ( 0.5625000000000000000, 0.5694444444444444198, 0.5833333333333333703, 0.5972222222222222099, 0.6041666666666665186 ),
 .UNSPECIFIED. ) 
 CURVE ( )  GEOMETRIC_REPRESENTATION_ITEM ( )  RATIONAL_B_SPLINE_CURVE ( ( 0.9330127018922194093, 0.9330127018922194093, 1.000000000000000000, 0.8660254037844387076, 1.000000000000000000, 0.8660254037844387076, 1.000000000000000000, 0.9330127018922209636, 0.9330127018922194093 ) ) 
 REPRESENTATION_ITEM ( '' )  );
#4039=CARTESIAN_POINT ( 'NONE',  ( -85.15643035624999868, -34.34062499938548285, 98.40857419181659793 ) ) ;
#4043=CARTESIAN_POINT ( 'NONE',  ( -85.15643035624999868, -34.15312499938548285, 101.5914258081833879 ) ) ;
#4049=CARTESIAN_POINT ( 'NONE',  ( -79.64356964374998427, -35.01562499938548711, 101.5914258081833879 ) ) ;
#4059=CARTESIAN_POINT ( 'NONE',  ( -79.39999999999999147, -34.68750000000000000, 98.26794919243110371 ) ) ;
#4081=CYLINDRICAL_SURFACE ( 'NONE', #580, 3.000000000000002665 ) ;
#4085=CARTESIAN_POINT ( 'NONE',  ( -82.40000000000000568, -30.00000000000000355, 99.99999999999998579 ) ) ;
#4090=CARTESIAN_POINT ( 'NONE',  ( -85.40000000000000568, -34.46249999999999858, 101.7320508075688821 ) ) ;
#4091=CARTESIAN_POINT ( 'NONE',  ( -82.39999999999999147, -34.78124999877096712, 103.4641016151377499 ) ) ;
#4092=CARTESIAN_POINT ( 'NONE',  ( -85.15643035624999868, -31.19062499938548783, 98.40857419181659793 ) ) ;
#4105=CARTESIAN_POINT ( 'NONE',  ( -82.65380294351676582, -34.99990492518305274, 97.01075526832239859 ) ) ;
#4106=CARTESIAN_POINT ( 'NONE',  ( -82.39999999999999147, -31.60312499938548569, 96.81714838363319586 ) ) ;
#4117=CARTESIAN_POINT ( 'NONE',  ( -85.40000000000000568, -31.80000000000000071, 99.99999999999998579 ) ) ;
#4132=CARTESIAN_POINT ( 'NONE',  ( -83.77821517812500929, -33.92812499938548854, 97.61286128772489690 ) ) ;
#4136=CARTESIAN_POINT ( 'NONE',  ( -85.15643035625001289, -33.29062499938547859, 99.99999999999998579 ) ) ;
#4152=ORIENTED_EDGE ( 'NONE', *, *, #10678, .T. ) ;
#4156=CARTESIAN_POINT ( 'NONE',  ( -85.40000000000000568, -33.60000000000000142, 99.99999999999998579 ) ) ;
#4183=ORIENTED_EDGE ( 'NONE', *, *, #9647, .F. ) ;
#4188=CARTESIAN_POINT ( 'NONE',  ( -83.90000000000000568, -34.81874999877096855, 102.5980762113533018 ) ) ;
#4189=CARTESIAN_POINT ( 'NONE',  ( -85.15643035625001289, -31.15312499938548996, 99.99999999999998579 ) ) ;
#4200=CARTESIAN_POINT ( 'NONE',  ( -81.02178482187500208, -32.09062499938548285, 97.61286128772489690 ) ) ;
#4212=CARTESIAN_POINT ( 'NONE',  ( -80.90000000000000568, -31.20000000000000284, 102.5980762113533018 ) ) ;
#4214=CARTESIAN_POINT ( 'NONE',  ( -84.51155153715826884, -35.14114847181267720, 98.22820474807231506 ) ) ;
#4221=DIRECTION ( 'NONE',  ( -0.000000000000000000, -1.000000000000000000, -0.000000000000000000 ) ) ;
#4227=CARTESIAN_POINT ( 'NONE',  ( -85.15643035624999868, -31.90312499938548285, 101.5914258081833879 ) ) ;
#4228=CARTESIAN_POINT ( 'NONE',  ( -85.40000000000000568, -34.01250000000000284, 101.7320508075688821 ) ) ;
#4233=CARTESIAN_POINT ( 'NONE',  ( -82.39999999999999147, -34.75312499938549138, 96.81714838363319586 ) ) ;
#4241=CARTESIAN_POINT ( 'NONE',  ( -81.59615242270662350, -30.76740381056766793, 102.9999999999999858 ) ) ;
#4244=B_SPLINE_CURVE_WITH_KNOTS ( 'NONE', 3,
 ( #4105, #9778, #18770, #18867, #4013, #8308 ),
 .UNSPECIFIED., .F., .F.,
 ( 4, 2, 4 ),
 ( 0.5134810729395012929, 0.5761852797268253168, 0.6388894865141493407 ),
 .UNSPECIFIED. ) ;
#4251=CARTESIAN_POINT ( 'NONE',  ( -85.39999999999999147, -34.97364041986484295, 98.90809577818232867 ) ) ;
#4255=CARTESIAN_POINT ( 'NONE',  ( -85.40000000000000568, -30.48749999999999716, 98.26794919243111792 ) ) ;
#4258=CARTESIAN_POINT ( 'NONE',  ( -79.39999999999999147, -33.37106250001229313, 99.99999999999998579 ) ) ;
#4260=EDGE_CURVE ( 'NONE', #17075, #2327, #9355, .T. ) ;
#4262=CARTESIAN_POINT ( 'NONE',  ( -83.77821517812500929, -31.56562499938548427, 97.61286128772489690 ) ) ;
#4275=VERTEX_POINT ( 'NONE', #10852 ) ;
#4285=CARTESIAN_POINT ( 'NONE',  ( -82.39999999999999147, -33.43124999877097281, 103.4641016151377499 ) ) ;
#4287=CARTESIAN_POINT ( 'NONE',  ( -79.64356964374999848, -33.62812499938548427, 99.99999999999998579 ) ) ;
#4288=CARTESIAN_POINT ( 'NONE',  ( -80.90000000000000568, -31.65000000000000568, 102.5980762113533018 ) ) ;
#4298=CARTESIAN_POINT ( 'NONE',  ( -83.77821517812500929, -34.11562499938548854, 102.3871387122750889 ) ) ;
#4305=ORIENTED_EDGE ( 'NONE', *, *, #8001, .F. ) ;
#4306=CARTESIAN_POINT ( 'NONE',  ( -83.90000000000000568, -31.66874999877096997, 102.5980762113533018 ) ) ;
#4312=CARTESIAN_POINT ( 'NONE',  ( -85.40000000000000568, -32.66250000000000142, 101.7320508075688679 ) ) ;
#4313=FACE_OUTER_BOUND ( 'NONE', #6565, .T. ) ;
#4326=CARTESIAN_POINT ( 'NONE',  ( -83.77821517812500929, -30.21562499938548285, 97.61286128772489690 ) ) ;
#4330=ORIENTED_EDGE ( 'NONE', *, *, #9496, .T. ) ;
#4332=CARTESIAN_POINT ( 'NONE',  ( -85.40000000000000568, -30.45000000000000284, 99.99999999999998579 ) ) ;
#4342=CARTESIAN_POINT ( 'NONE',  ( -81.59615242270662350, -31.42634618820330772, 97.00000000000000000 ) ) ;
#4353=CARTESIAN_POINT ( 'NONE',  ( -79.39999999999999147, -31.60856250001229029, 101.7320508075688537 ) ) ;
#4358=CARTESIAN_POINT ( 'NONE',  ( -81.02178482187500208, -32.24062499938548854, 102.3871387122750889 ) ) ;
#4377=CARTESIAN_POINT ( 'NONE',  ( -83.20384757729335945, -32.28615380933863577, 97.00000000000000000 ) ) ;
#4382=CARTESIAN_POINT ( 'NONE',  ( -83.90000000000000568, -32.12268749875867968, 102.5980762113533018 ) ) ;
#4383=CARTESIAN_POINT ( 'NONE',  ( -79.64356964375001269, -34.11562499938548854, 101.5914258081833879 ) ) ;
#4394=CARTESIAN_POINT ( 'NONE',  ( -79.64356964374999848, -33.51562499938548711, 99.99999999999998579 ) ) ;
#4395=ORIENTED_EDGE ( 'NONE', *, *, #5417, .F. ) ;
#4406=CARTESIAN_POINT ( 'NONE',  ( -82.39999999999999147, -32.58750000000000568, 103.4641016151377499 ) ) ;
#4407=CARTESIAN_POINT ( 'NONE',  ( -79.39999999999999147, -31.96874999877096712, 99.99999999999998579 ) ) ;
#4418=CARTESIAN_POINT ( 'NONE',  ( -83.77821517812500929, -30.51562499938548711, 102.3871387122750889 ) ) ;
#4424=CARTESIAN_POINT ( 'NONE',  ( -79.39999999999999147, -31.08750000000000213, 98.26794919243110371 ) ) ;
#4445=AXIS2_PLACEMENT_3D ( 'NONE', #1671, #10745, #11831 ) ;
#4449=CARTESIAN_POINT ( 'NONE',  ( -79.39999999999999147, -32.05856250001228602, 101.7320508075688537 ) ) ;
#4450=EDGE_CURVE ( 'NONE', #16779, #9677, #18256, .T. ) ;
#4454=CARTESIAN_POINT ( 'NONE',  ( -79.64356964375001269, -31.22812499938548925, 98.40857419181659793 ) ) ;
#4461=ORIENTED_EDGE ( 'NONE', *, *, #11966, .T. ) ;
#4477=CARTESIAN_POINT ( 'NONE',  ( -82.39999999999999147, -30.96018749875868181, 96.53589838486223584 ) ) ;
#4478=CARTESIAN_POINT ( 'NONE',  ( -79.64356964374999848, -34.07812499938548711, 99.99999999999998579 ) ) ;
#4479=CARTESIAN_POINT ( 'NONE',  ( -81.59615242270660929, -31.48259618943233207, 96.99999999999997158 ) ) ;
#4490=CARTESIAN_POINT ( 'NONE',  ( -85.15643035625001289, -34.60312499938548569, 101.5914258081833879 ) ) ;
#4494=CARTESIAN_POINT ( 'NONE',  ( -84.70833260042415702, -35.00006955123599539, 98.08383195543535749 ) ) ;
#4501=CARTESIAN_POINT ( 'NONE',  ( -82.39999999999999147, -34.38750000000000284, 103.4641016151377499 ) ) ;
#4502=CARTESIAN_POINT ( 'NONE',  ( -85.40000000000000568, -30.80624999877096926, 101.7320508075688679 ) ) ;
#4513=CARTESIAN_POINT ( 'NONE',  ( -79.64356964375001269, -30.32812499938548711, 98.40857419181659793 ) ) ;
#4519=CARTESIAN_POINT ( 'NONE',  ( -82.39999999999999147, -30.33750000000000213, 103.4641016151377499 ) ) ;
#4528=VECTOR ( 'NONE', #14030, 1000.000000000000000 ) ;
#4544=CARTESIAN_POINT ( 'NONE',  ( -82.40000000000000568, -30.00000000000000355, 96.99999999999998579 ) ) ;
#4546=CARTESIAN_POINT ( 'NONE',  ( -80.90000000000000568, -31.64606250001229881, 102.5980762113533018 ) ) ;
#4549=CARTESIAN_POINT ( 'NONE',  ( -85.15643035624999868, -32.42812499938548854, 98.40857419181659793 ) ) ;
#4560=CARTESIAN_POINT ( 'NONE',  ( -82.40000000000000568, -33.03750000000000142, 102.9999999999999858 ) ) ;
#4571=CARTESIAN_POINT ( 'NONE',  ( -85.40000000000000568, -32.68518749875868679, 98.26794919243111792 ) ) ;
#4572=CARTESIAN_POINT ( 'NONE',  ( -85.15643035624999868, -32.99062499938548854, 98.40857419181659793 ) ) ;
#4578=( BOUNDED_CURVE ( )  B_SPLINE_CURVE ( 2, ( #8749, #11780, #2692, #13239, #14608, #8649, #17650, #11398, #10128 ),
 .UNSPECIFIED., .F., .F. ) 
 B_SPLINE_CURVE_WITH_KNOTS ( ( 3, 2, 2, 2, 3 ),
 ( 0.3958333333333334259, 0.4027777777777777901, 0.4166666666666666852, 0.4305555555555555802, 0.4374999999999999445 ),
 .UNSPECIFIED. ) 
 CURVE ( )  GEOMETRIC_REPRESENTATION_ITEM ( )  RATIONAL_B_SPLINE_CURVE ( ( 0.9330127018922192983, 0.9330127018922200755, 1.000000000000000000, 0.8660254037844387076, 1.000000000000000000, 0.8660254037844387076, 1.000000000000000000, 0.9330127018922198534, 0.9330127018922192983 ) ) 
 REPRESENTATION_ITEM ( '' )  );
#4579=CARTESIAN_POINT ( 'NONE',  ( -82.40000000000000568, -30.11250000000000071, 96.99999999999998579 ) ) ;
#4589=CARTESIAN_POINT ( 'NONE',  ( -82.39999999999999147, -32.72812499938548569, 103.1828516163667899 ) ) ;
#4590=ORIENTED_EDGE ( 'NONE', *, *, #6653, .F. ) ;
#4600=CARTESIAN_POINT ( 'NONE',  ( -85.40000000000000568, -34.91250000000000142, 101.7320508075688679 ) ) ;
#4602=CARTESIAN_POINT ( 'NONE',  ( -83.90000000000000568, -32.26874999877097139, 97.40192378864668399 ) ) ;
#4616=CARTESIAN_POINT ( 'NONE',  ( -83.77821517812500929, -30.96562499938548640, 102.3871387122750889 ) ) ;
#4623=CARTESIAN_POINT ( 'NONE',  ( -82.39999999999999147, -31.91249999999999787, 96.99999999999998579 ) ) ;
#4625=CARTESIAN_POINT ( 'NONE',  ( -85.40000000000000568, -30.00000000000000355, 99.99999999999998579 ) ) ;
#4633=CYLINDRICAL_SURFACE ( 'NONE', #10867, 3.000000000000002665 ) ;
#4651=CARTESIAN_POINT ( 'NONE',  ( -85.40000000000000568, -33.14606250001229171, 99.99999999999998579 ) ) ;
#4658=CARTESIAN_POINT ( 'NONE',  ( -82.40000000000000568, -30.00000000000000355, 96.99999999999998579 ) ) ;
#4665=( BOUNDED_CURVE ( )  B_SPLINE_CURVE ( 2, ( #11953, #4342, #13223, #6204, #14786, #9025, #245, #12152, #14985 ),
 .UNSPECIFIED., .F., .F. ) 
 B_SPLINE_CURVE_WITH_KNOTS ( ( 3, 2, 2, 2, 3 ),
 ( 0.1875000000000000278, 0.1944444444444444475, 0.2083333333333333426, 0.2222222222222222099, 0.2291666666666666574 ),
 .UNSPECIFIED. ) 
 CURVE ( )  GEOMETRIC_REPRESENTATION_ITEM ( )  RATIONAL_B_SPLINE_CURVE ( ( 0.9330127018922194093, 0.9330127018922196314, 1.000000000000000000, 0.8660254037844387076, 1.000000000000000000, 0.8660254037844387076, 1.000000000000000000, 0.9330127018922194093, 0.9330127018922194093 ) ) 
 REPRESENTATION_ITEM ( '' )  );
#4667=EDGE_LOOP ( 'NONE', ( #5538, #3499, #17491, #1307 ) ) ;
#4674=CARTESIAN_POINT ( 'NONE',  ( -79.39999999999999147, -31.07268749875867897, 99.99999999999998579 ) ) ;
#4675=CARTESIAN_POINT ( 'NONE',  ( -83.77821517812500929, -34.37812499938548427, 97.61286128772489690 ) ) ;
#4686=CARTESIAN_POINT ( 'NONE',  ( -85.15643035625001289, -33.74062499938548854, 99.99999999999998579 ) ) ;
#4693=DIRECTION ( 'NONE',  ( 0.000000000000000000, -1.000000000000000000, 0.000000000000000000 ) ) ;
#4697=CARTESIAN_POINT ( 'NONE',  ( -85.40000000000000568, -33.56250000000000000, 101.7320508075688679 ) ) ;
#4699=CARTESIAN_POINT ( 'NONE',  ( -85.40000000000000568, -31.70624999877096784, 101.7320508075688679 ) ) ;
#4710=( NAMED_UNIT ( * ) SI_UNIT ( $, .STERADIAN. ) SOLID_ANGLE_UNIT ( ) );
#4715=FACE_OUTER_BOUND ( 'NONE', #16745, .T. ) ;
#4721=CARTESIAN_POINT ( 'NONE',  ( -80.90000000000000568, -31.50000000000000000, 97.40192378864668399 ) ) ;
#4738=CARTESIAN_POINT ( 'NONE',  ( -82.39999999999999147, -31.04062499938548569, 103.1828516163667899 ) ) ;
#4742=CARTESIAN_POINT ( 'NONE',  ( -79.50134204033872720, -34.99892421733355263, 100.8484099402798222 ) ) ;
#4745=CARTESIAN_POINT ( 'NONE',  ( -82.39999999999999147, -32.58750000000000568, 102.9999999999999858 ) ) ;
#4746=CARTESIAN_POINT ( 'NONE',  ( -85.40000000000000568, -30.90000000000000213, 99.99999999999998579 ) ) ;
#4751=CARTESIAN_POINT ( 'NONE',  ( -79.64356964374998427, -32.31562499938548427, 101.5914258081833879 ) ) ;
#4759=PRODUCT_DEFINITION_CONTEXT ( 'detailed design', #17572, 'design' ) ;
#4763=VECTOR ( 'NONE', #6791, 1000.000000000000000 ) ;
#4770=CARTESIAN_POINT ( 'NONE',  ( -82.39999999999999147, -32.30624999877096570, 96.99999999999998579 ) ) ;
#4775=CARTESIAN_POINT ( 'NONE',  ( -80.90000000000000568, -31.89768749875867471, 97.40192378864668399 ) ) ;
#4802=CARTESIAN_POINT ( 'NONE',  ( -81.59615242270662350, -33.73259618943233562, 96.99999999999998579 ) ) ;
#4803=CARTESIAN_POINT ( 'NONE',  ( -79.39999999999999147, -30.65624999877096712, 101.7320508075688537 ) ) ;
#4804=CARTESIAN_POINT ( 'NONE',  ( -85.40000000000000568, -32.60624999877097707, 101.7320508075688679 ) ) ;
#4814=CARTESIAN_POINT ( 'NONE',  ( -82.40000000000001990, -33.93750000000000711, 103.0000000000000000 ) ) ;
#4836=CARTESIAN_POINT ( 'NONE',  ( -83.77821517812500929, -30.77812499938548640, 97.61286128772489690 ) ) ;
#4839=EDGE_CURVE ( 'NONE', #12897, #6852, #9299, .T. ) ;
#4844=CARTESIAN_POINT ( 'NONE',  ( -83.77821517812500929, -31.97812499938548925, 102.3871387122750889 ) ) ;
#4855=AXIS2_PLACEMENT_3D ( 'NONE', #6523, #2302, #9536 ) ;
#4859=ORIENTED_EDGE ( 'NONE', *, *, #2361, .F. ) ;
#4867=CARTESIAN_POINT ( 'NONE',  ( -85.40000000000000568, -34.89768749875867826, 99.99999999999998579 ) ) ;
#4892=CARTESIAN_POINT ( 'NONE',  ( -80.90000000000000568, -34.20000000000000284, 97.40192378864668399 ) ) ;
#4893=CARTESIAN_POINT ( 'NONE',  ( -80.90000000000000568, -34.35000000000000853, 102.5980762113533018 ) ) ;
#4894=CARTESIAN_POINT ( 'NONE',  ( -85.40000000000000568, -33.05624999877096570, 101.7320508075688679 ) ) ;
#4906=CARTESIAN_POINT ( 'NONE',  ( -85.15643035625001289, -30.25312499938548783, 99.99999999999998579 ) ) ;
#4909=VERTEX_POINT ( 'NONE', #2009 ) ;
#4918=CARTESIAN_POINT ( 'NONE',  ( -82.40000000000000568, -50.00000000000000000, 99.99999999999998579 ) ) ;
#4921=ADVANCED_FACE ( 'NONE', ( #3280 ), #13924, .T. ) ;
#4932=CARTESIAN_POINT ( 'NONE',  ( -83.77821517812500929, -32.42812499938548854, 102.3871387122750889 ) ) ;
#4942=CARTESIAN_POINT ( 'NONE',  ( -82.39999999999999147, -31.94062499938548427, 103.1828516163667899 ) ) ;
#4968=CARTESIAN_POINT ( 'NONE',  ( -80.90000000000000568, -34.14768749875867826, 97.40192378864668399 ) ) ;
#4972=CARTESIAN_POINT ( 'NONE',  ( -82.39999999999999147, -34.33124999877097139, 103.0000000000000000 ) ) ;
#4983=CARTESIAN_POINT ( 'NONE',  ( -85.15643035624999868, -34.22812499938547859, 98.40857419181659793 ) ) ;
#4984=CARTESIAN_POINT ( 'NONE',  ( -82.39999999999999147, -34.75312499938548427, 96.81714838363319586 ) ) ;
#4994=CARTESIAN_POINT ( 'NONE',  ( -85.40000000000000568, -32.60624999877097707, 101.7320508075688679 ) ) ;
#4996=CARTESIAN_POINT ( 'NONE',  ( -79.39999999999999147, -32.90624999877096712, 101.7320508075688537 ) ) ;
#5002=( LENGTH_UNIT ( ) NAMED_UNIT ( * ) SI_UNIT ( .MILLI., .METRE. ) );
#5007=CARTESIAN_POINT ( 'NONE',  ( -82.40000000000000568, -33.65624999877097423, 97.00000000000000000 ) ) ;
#5029=CARTESIAN_POINT ( 'NONE',  ( -85.15643035624999868, -32.46562499938548996, 101.5914258081833879 ) ) ;
#5033=CARTESIAN_POINT ( 'NONE',  ( -85.11055541976942607, -34.99883777075648084, 98.66815749044441475 ) ) ;
#5037=CARTESIAN_POINT ( 'NONE',  ( -83.77821517812500929, -30.77812499938548640, 97.61286128772489690 ) ) ;
#5054=EDGE_CURVE ( 'NONE', #2550, #8815, #5143, .T. ) ;
#5059=CARTESIAN_POINT ( 'NONE',  ( -79.39999999999999147, -33.73518749875868394, 98.26794919243110371 ) ) ;
#5061=LINE ( 'NONE', #11099, #17114 ) ;
#5062=CARTESIAN_POINT ( 'NONE',  ( -85.40000000000000568, -34.40624999877096712, 101.7320508075688821 ) ) ;
#5068=AXIS2_PLACEMENT_3D ( 'NONE', #13206, #1492, #13020 ) ;
#5076=CARTESIAN_POINT ( 'NONE',  ( -81.02178482187500208, -32.54062499938548569, 97.61286128772489690 ) ) ;
#5079=ORIENTED_EDGE ( 'NONE', *, *, #6126, .F. ) ;
#5086=CARTESIAN_POINT ( 'NONE',  ( -79.39999999999999147, -34.23750000000000426, 98.26794919243110371 ) ) ;
#5087=CARTESIAN_POINT ( 'NONE',  ( -83.90000000000000568, -32.56874999877096855, 102.5980762113533018 ) ) ;
#5088=CARTESIAN_POINT ( 'NONE',  ( -79.39999999999999147, -35.15624999877096712, 101.7320508075688537 ) ) ;
#5098=AXIS2_PLACEMENT_3D ( 'NONE', #2939, #19264, #15144 ) ;
#5100=CARTESIAN_POINT ( 'NONE',  ( -85.40000000000000568, -33.54374999877096286, 99.99999999999998579 ) ) ;
#5112=CARTESIAN_POINT ( 'NONE',  ( -79.39999999999999147, -34.23356250001229739, 98.26794919243110371 ) ) ;
#5113=EDGE_CURVE ( 'NONE', #15126, #12906, #12145, .T. ) ;
#5124=CARTESIAN_POINT ( 'NONE',  ( -81.02178482187500208, -31.00312499938548783, 102.3871387122750889 ) ) ;
#5127=ORIENTED_EDGE ( 'NONE', *, *, #17486, .F. ) ;
#5132=CARTESIAN_POINT ( 'NONE',  ( -85.15643035625001289, -31.19062499938548783, 98.40857419181659793 ) ) ;
#5139=ORIENTED_EDGE ( 'NONE', *, *, #16654, .T. ) ;
#5143=LINE ( 'NONE', #11385, #16797 ) ;
#5147=CARTESIAN_POINT ( 'NONE',  ( -81.59615242270663771, -32.51115380933863008, 103.0000000000000000 ) ) ;
#5151=CARTESIAN_POINT ( 'NONE',  ( -79.39999999999999147, -35.12268749875867258, 99.99999999999998579 ) ) ;
#5153=CARTESIAN_POINT ( 'NONE',  ( -83.77821517812500929, -35.12812499938548427, 102.3871387122750889 ) ) ;
#5161=ORIENTED_EDGE ( 'NONE', *, *, #54, .T. ) ;
#5166=CARTESIAN_POINT ( 'NONE',  ( -81.02178482187500208, -33.14062499938548711, 102.3871387122750889 ) ) ;
#5175=VECTOR ( 'NONE', #12765, 1000.000000000000000 ) ;
#5178=CARTESIAN_POINT ( 'NONE',  ( -83.90000000000000568, -31.66874999877096997, 102.5980762113533018 ) ) ;
#5179=( BOUNDED_CURVE ( )  B_SPLINE_CURVE ( 2, ( #7944, #636, #16740, #9310, #6490, #13896, #15273, #7847, #10874 ),
 .UNSPECIFIED., .F., .F. ) 
 B_SPLINE_CURVE_WITH_KNOTS ( ( 3, 2, 2, 2, 3 ),
 ( 0.1458333333333333426, 0.1527777777777777901, 0.1666666666666666574, 0.1805555555555555525, 0.1875000000000000000 ),
 .UNSPECIFIED. ) 
 CURVE ( )  GEOMETRIC_REPRESENTATION_ITEM ( )  RATIONAL_B_SPLINE_CURVE ( ( 0.9330127018922194093, 0.9330127018922194093, 1.000000000000000000, 0.8660254037844387076, 1.000000000000000000, 0.8660254037844387076, 1.000000000000000000, 0.9330127018922194093, 0.9330127018922194093 ) ) 
 REPRESENTATION_ITEM ( '' )  );
#5180=CARTESIAN_POINT ( 'NONE',  ( -85.40000000000000568, -33.99374999877097281, 99.99999999999998579 ) ) ;
#5196=CARTESIAN_POINT ( 'NONE',  ( -82.39999999999999147, -31.85624999877096641, 96.99999999999998579 ) ) ;
#5197=CARTESIAN_POINT ( 'NONE',  ( -81.59615242270662350, -33.67634618820330417, 96.99999999999997158 ) ) ;
#5206=CARTESIAN_POINT ( 'NONE',  ( -85.40000000000000568, -34.49606250001229313, 99.99999999999998579 ) ) ;
#5219=CARTESIAN_POINT ( 'NONE',  ( -79.64356964375001269, -33.21562499938548996, 101.5914258081833879 ) ) ;
#5223=EDGE_LOOP ( 'NONE', ( #11320, #18728, #3955, #9066, #3118, #4395 ) ) ;
#5231=CARTESIAN_POINT ( 'NONE',  ( -85.15643035625001289, -33.89062499938548711, 98.40857419181659793 ) ) ;
#5242=CARTESIAN_POINT ( 'NONE',  ( -79.39999999999999147, -32.47500000000000142, 99.99999999999998579 ) ) ;
#5253=CARTESIAN_POINT ( 'NONE',  ( -82.39999999999999147, -30.55856250001229668, 96.53589838486223584 ) ) ;
#5255=CARTESIAN_POINT ( 'NONE',  ( -80.90000000000000568, -34.29768749875867684, 102.5980762113533018 ) ) ;
#5257=B_SPLINE_CURVE_WITH_KNOTS ( 'NONE', 1,
 ( #805, #14171 ),
 .UNSPECIFIED., .F., .F.,
 ( 2, 2 ),
 ( 0.000000000000000000, 1.000000000000000000 ),
 .UNSPECIFIED. ) ;
#5259=CARTESIAN_POINT ( 'NONE',  ( -85.15643035625001289, -30.14062499938548711, 99.99999999999998579 ) ) ;
#5272=CARTESIAN_POINT ( 'NONE',  ( -79.64356964374999848, -32.61562499938548854, 99.99999999999998579 ) ) ;
#5282=CARTESIAN_POINT ( 'NONE',  ( -79.39999999999999147, -31.10624999877097352, 101.7320508075688537 ) ) ;
#5283=CARTESIAN_POINT ( 'NONE',  ( -82.39999999999999147, -34.78124999877096712, 103.4641016151377499 ) ) ;
#5295=CARTESIAN_POINT ( 'NONE',  ( -79.64356964374998427, -32.20312499938548711, 101.5914258081833879 ) ) ;
#5309=CARTESIAN_POINT ( 'NONE',  ( -85.40000000000000568, -30.41249999999999787, 101.7320508075688679 ) ) ;
#5311=DIRECTION ( 'NONE',  ( 0.000000000000000000, -1.000000000000000000, 0.000000000000000000 ) ) ;
#5314=CARTESIAN_POINT ( 'NONE',  ( -81.59615242270662350, -33.46740381056766722, 102.9999999999999716 ) ) ;
#5321=LINE ( 'NONE', #14378, #9896 ) ;
#5323=CARTESIAN_POINT ( 'NONE',  ( -85.15643035625001289, -32.95312499938548711, 99.99999999999998579 ) ) ;
#5329=CARTESIAN_POINT ( 'NONE',  ( -79.64356964375001269, -33.55312499938548854, 101.5914258081833879 ) ) ;
#5335=( BOUNDED_CURVE ( )  B_SPLINE_CURVE ( 2, ( #521, #6474, #3726, #811, #17019 ),
 .UNSPECIFIED., .F., .F. ) 
 B_SPLINE_CURVE_WITH_KNOTS ( ( 3, 2, 3 ),
 ( 0.000000000000000000, 0.01388888888888888638, 0.02083333333333331136 ),
 .UNSPECIFIED. ) 
 CURVE ( )  GEOMETRIC_REPRESENTATION_ITEM ( )  RATIONAL_B_SPLINE_CURVE ( ( 1.000000000000000000, 0.8660254037844387076, 1.000000000000000000, 0.9330127018922196314, 0.9330127018922194093 ) ) 
 REPRESENTATION_ITEM ( '' )  );
#5336=CARTESIAN_POINT ( 'NONE',  ( -83.77821517812500929, -33.77812499938548285, 102.3871387122750889 ) ) ;
#5345=CARTESIAN_POINT ( 'NONE',  ( -80.90000000000000568, -33.75000000000000000, 97.40192378864668399 ) ) ;
#5357=CARTESIAN_POINT ( 'NONE',  ( -85.15643035624999868, -30.17812499938548498, 98.40857419181659793 ) ) ;
#5368=CARTESIAN_POINT ( 'NONE',  ( -79.64356964375001269, -32.65312499938548285, 101.5914258081833879 ) ) ;
#5372=DIRECTION ( 'NONE',  ( -0.000000000000000000, -1.000000000000000000, -0.000000000000000000 ) ) ;
#5378=CARTESIAN_POINT ( 'NONE',  ( -83.90000000000000568, -31.21874999877097068, 102.5980762113533018 ) ) ;
#5379=CARTESIAN_POINT ( 'NONE',  ( -81.02178482187500208, -31.90312499938548996, 102.3871387122750889 ) ) ;
#5382=VECTOR ( 'NONE', #15745, 1000.000000000000000 ) ;
#5393=CARTESIAN_POINT ( 'NONE',  ( -79.64356964374999848, -31.26562499938548356, 99.99999999999998579 ) ) ;
#5406=CARTESIAN_POINT ( 'NONE',  ( -82.39999999999999147, -30.78750000000000497, 103.4641016151377499 ) ) ;
#5417=EDGE_CURVE ( 'NONE', #7672, #16645, #2784, .T. ) ;
#5421=CARTESIAN_POINT ( 'NONE',  ( -82.39999999999999147, -34.19062499938548427, 103.1828516163667899 ) ) ;
#5425=CARTESIAN_POINT ( 'NONE',  ( -81.02178482187500208, -33.44062499938548427, 97.61286128772489690 ) ) ;
#5427=( BOUNDED_CURVE ( )  B_SPLINE_CURVE ( 2, ( #18561, #13959, #15330, #9670, #16706, #9469, #15631, #12593, #601 ),
 .UNSPECIFIED., .F., .F. ) 
 B_SPLINE_CURVE_WITH_KNOTS ( ( 3, 2, 2, 2, 3 ),
 ( 0.3541666666666666852, 0.3611111111111111049, 0.3750000000000000000, 0.3888888888888888951, 0.3958333333333334259 ),
 .UNSPECIFIED. ) 
 CURVE ( )  GEOMETRIC_REPRESENTATION_ITEM ( )  RATIONAL_B_SPLINE_CURVE ( ( 0.9330127018922194093, 0.9330127018922196314, 1.000000000000000000, 0.8660254037844387076, 1.000000000000000000, 0.8660254037844387076, 1.000000000000000000, 0.9330127018922185211, 0.9330127018922192983 ) ) 
 REPRESENTATION_ITEM ( '' )  );
#5433=CARTESIAN_POINT ( 'NONE',  ( -81.02178482187500208, -34.45312499938548711, 97.61286128772489690 ) ) ;
#5444=CARTESIAN_POINT ( 'NONE',  ( -80.90000000000000568, -34.64999999999999858, 97.40192378864668399 ) ) ;
#5447=CARTESIAN_POINT ( 'NONE',  ( -82.39999999999999147, -31.23750000000000071, 102.9999999999999858 ) ) ;
#5452=CARTESIAN_POINT ( 'NONE',  ( -80.90000000000000568, -31.04606250001229029, 97.40192378864668399 ) ) ;
#5454=CARTESIAN_POINT ( 'NONE',  ( -82.40000000000000568, -30.00000000000000355, 99.99999999999998579 ) ) ;
#5468=ORIENTED_EDGE ( 'NONE', *, *, #13152, .T. ) ;
#5471=CARTESIAN_POINT ( 'NONE',  ( -82.40000000000000568, -30.00000000000000355, 96.99999999999998579 ) ) ;
#5476=CARTESIAN_POINT ( 'NONE',  ( -82.40000000000000568, -34.38749999999999574, 102.9999999999999858 ) ) ;
#5477=CARTESIAN_POINT ( 'NONE',  ( -85.40000000000000568, -35.34374999877096712, 99.99999999999998579 ) ) ;
#5478=CARTESIAN_POINT ( 'NONE',  ( -83.77821517812500929, -31.22812499938548569, 97.61286128772489690 ) ) ;
#5490=CARTESIAN_POINT ( 'NONE',  ( -79.64356964374999848, -32.16562499938548569, 99.99999999999998579 ) ) ;
#5501=CARTESIAN_POINT ( 'NONE',  ( -83.90000000000000568, -33.22500000000000142, 97.40192378864668399 ) ) ;
#5502=DIRECTION ( 'NONE',  ( -0.000000000000000000, -1.000000000000000000, -0.000000000000000000 ) ) ;
#5503=CARTESIAN_POINT ( 'NONE',  ( -82.40000000000000568, -30.00000000000000355, 99.99999999999998579 ) ) ;
#5511=DIRECTION ( 'NONE',  ( 0.000000000000000000, 0.000000000000000000, -1.000000000000000000 ) ) ;
#5514=CARTESIAN_POINT ( 'NONE',  ( -85.15643035625001289, -33.85312499938549280, 99.99999999999998579 ) ) ;
#5517=CARTESIAN_POINT ( 'NONE',  ( -79.64356964375001269, -34.37812499938548427, 98.40857419181659793 ) ) ;
#5521=CARTESIAN_POINT ( 'NONE',  ( -82.39999999999999147, -32.81250000000000000, 97.00000000000000000 ) ) ;
#5523=CARTESIAN_POINT ( 'NONE',  ( -81.02178482187500208, -33.25312499938548427, 102.3871387122750889 ) ) ;
#5533=CARTESIAN_POINT ( 'NONE',  ( -79.39999999999999147, -34.31250000000000000, 101.7320508075688537 ) ) ;
#5538=ORIENTED_EDGE ( 'NONE', *, *, #13776, .F. ) ;
#5541=EDGE_CURVE ( 'NONE', #6725, #3433, #7696, .T. ) ;
#5544=CARTESIAN_POINT ( 'NONE',  ( -80.90000000000000568, -31.19606250001229242, 102.5980762113533018 ) ) ;
#5548=CARTESIAN_POINT ( 'NONE',  ( -82.39999999999999147, -30.47812499938548569, 103.1828516163667899 ) ) ;
#5561=EDGE_CURVE ( 'NONE', #7994, #6852, #15867, .T. ) ;
#5567=LINE ( 'NONE', #5471, #2553 ) ;
#5574=CARTESIAN_POINT ( 'NONE',  ( -80.90000000000000568, -30.54768749875868039, 97.40192378864668399 ) ) ;
#5575=CARTESIAN_POINT ( 'NONE',  ( -81.02178482187500208, -30.55312499938548854, 102.3871387122750889 ) ) ;
#5586=CARTESIAN_POINT ( 'NONE',  ( -80.90000000000000568, -35.19374999877096855, 102.5980762113533018 ) ) ;
#5587=CARTESIAN_POINT ( 'NONE',  ( -79.64356964374998427, -31.75312499938548427, 101.5914258081833879 ) ) ;
#5599=CARTESIAN_POINT ( 'NONE',  ( -85.40000000000000568, -30.93750000000000355, 98.26794919243111792 ) ) ;
#5612=CARTESIAN_POINT ( 'NONE',  ( -82.39999999999999147, -34.64062499938548711, 103.1828516163667899 ) ) ;
#5616=CARTESIAN_POINT ( 'NONE',  ( -81.02178482187500208, -34.79062499938548569, 97.61286128772489690 ) ) ;
#5621=CARTESIAN_POINT ( 'NONE',  ( -85.15643035625001289, -33.81562499938548427, 101.5914258081833879 ) ) ;
#5631=CARTESIAN_POINT ( 'NONE',  ( -83.90000000000000568, -33.67500000000000426, 97.40192378864668399 ) ) ;
#5642=CARTESIAN_POINT ( 'NONE',  ( -83.90000000000000568, -33.67500000000000426, 97.40192378864668399 ) ) ;
#5654=EDGE_CURVE ( 'NONE', #8815, #6725, #2269, .T. ) ;
#5655=CARTESIAN_POINT ( 'NONE',  ( -85.15643035624999868, -35.05312499938548143, 101.5914258081833879 ) ) ;
#5657=ORIENTED_EDGE ( 'NONE', *, *, #6752, .F. ) ;
#5664=CARTESIAN_POINT ( 'NONE',  ( -85.40000000000000568, -34.50000000000000000, 99.99999999999998579 ) ) ;
#5665=CARTESIAN_POINT ( 'NONE',  ( -80.90000000000000568, -34.59374999877096712, 97.40192378864668399 ) ) ;
#5666=CARTESIAN_POINT ( 'NONE',  ( -82.39999999999999147, -32.16562499938549280, 96.81714838363319586 ) ) ;
#5680=CARTESIAN_POINT ( 'NONE',  ( -85.15643035625001289, -31.94062499938548427, 99.99999999999998579 ) ) ;
#5688=CARTESIAN_POINT ( 'NONE',  ( -79.39999999999999147, -31.12500000000000355, 99.99999999999998579 ) ) ;
#5690=CARTESIAN_POINT ( 'NONE',  ( -84.69814150944628750, -35.26302329524826007, 98.07164691963323833 ) ) ;
#5697=DIRECTION ( 'NONE',  ( -0.000000000000000000, -1.000000000000000000, -0.000000000000000000 ) ) ;
#5699=CARTESIAN_POINT ( 'NONE',  ( -81.02178482187500208, -31.64062499938548356, 97.61286128772489690 ) ) ;
#5700=CARTESIAN_POINT ( 'NONE',  ( -83.20384757729337366, -34.14240381056766438, 97.00000000000000000 ) ) ;
#5705=CARTESIAN_POINT ( 'NONE',  ( -81.02178482187500208, -34.34062499938548285, 97.61286128772489690 ) ) ;
#5709=CARTESIAN_POINT ( 'NONE',  ( -83.20384757729337366, -32.79240381056766296, 97.00000000000000000 ) ) ;
#5720=EDGE_CURVE ( 'NONE', #10587, #11600, #18768, .T. ) ;
#5730=CARTESIAN_POINT ( 'NONE',  ( -80.90000000000000568, -31.49606250001229313, 97.40192378864668399 ) ) ;
#5733=CARTESIAN_POINT ( 'NONE',  ( -85.15643035624999868, -31.00312499938548072, 101.5914258081833879 ) ) ;
#5734=CARTESIAN_POINT ( 'NONE',  ( -82.40000000000000568, -30.00000000000000355, 99.99999999999998579 ) ) ;
#5749=CARTESIAN_POINT ( 'NONE',  ( -82.39999999999999147, -32.30624999877096570, 96.99999999999998579 ) ) ;
#5754=CARTESIAN_POINT ( 'NONE',  ( -80.90000000000000568, -33.69374999877096855, 97.40192378864668399 ) ) ;
#5755=CARTESIAN_POINT ( 'NONE',  ( -79.64356964375001269, -32.31562499938548427, 101.5914258081833879 ) ) ;
#5765=CARTESIAN_POINT ( 'NONE',  ( -85.15643035625001289, -33.77812499938548285, 98.40857419181659793 ) ) ;
#5773=CARTESIAN_POINT ( 'NONE',  ( -85.40000000000000568, -31.70624999877096784, 101.7320508075688821 ) ) ;
#5777=CARTESIAN_POINT ( 'NONE',  ( -82.39999999999999147, -31.23750000000000071, 103.4641016151377499 ) ) ;
#5779=ADVANCED_FACE ( 'NONE', ( #18461 ), #15526, .T. ) ;
#5790=CARTESIAN_POINT ( 'NONE',  ( -82.39999999999999147, -30.47812499938548569, 103.1828516163667899 ) ) ;
#5791=CARTESIAN_POINT ( 'NONE',  ( -85.40000000000000568, -34.08749999999999858, 98.26794919243111792 ) ) ;
#5796=ORIENTED_EDGE ( 'NONE', *, *, #3028, .F. ) ;
#5798=CARTESIAN_POINT ( 'NONE',  ( -85.40000000000000568, -31.80000000000000071, 99.99999999999998579 ) ) ;
#5824=CARTESIAN_POINT ( 'NONE',  ( -83.90000000000000568, -33.22106250001229455, 97.40192378864668399 ) ) ;
#5825=EDGE_CURVE ( 'NONE', #10334, #6130, #15629, .T. ) ;
#5828=CARTESIAN_POINT ( 'NONE',  ( -81.02178482187500208, -31.19062499938548427, 97.61286128772489690 ) ) ;
#5852=CARTESIAN_POINT ( 'NONE',  ( -83.90000000000000568, -32.27268749875867115, 97.40192378864668399 ) ) ;
#5854=CARTESIAN_POINT ( 'NONE',  ( -85.15643035625001289, -33.40312499938548285, 99.99999999999998579 ) ) ;
#5866=CARTESIAN_POINT ( 'NONE',  ( -82.39999999999999147, -34.30312499938548143, 96.81714838363319586 ) ) ;
#5879=CARTESIAN_POINT ( 'NONE',  ( -85.40000000000000568, -31.38749999999999574, 98.26794919243111792 ) ) ;
#5880=CARTESIAN_POINT ( 'NONE',  ( -85.40000000000000568, -31.33124999877096428, 98.26794919243111792 ) ) ;
#5883=CARTESIAN_POINT ( 'NONE',  ( -84.69814120060431151, -35.16451018433117781, 98.07164655156650213 ) ) ;
#5892=CARTESIAN_POINT ( 'NONE',  ( -82.39999999999999147, -32.05312499938548854, 96.81714838363319586 ) ) ;
#5900=CARTESIAN_POINT ( 'NONE',  ( -83.90000000000000568, -31.42500000000000071, 97.40192378864668399 ) ) ;
#5910=EDGE_CURVE ( 'NONE', #1272, #16645, #5567, .T. ) ;
#5916=CARTESIAN_POINT ( 'NONE',  ( -85.40000000000000568, -34.95000000000000284, 99.99999999999998579 ) ) ;
#5923=CARTESIAN_POINT ( 'NONE',  ( -85.40000000000000568, -33.10856250001229739, 101.7320508075688679 ) ) ;
#5926=CARTESIAN_POINT ( 'NONE',  ( -82.39999999999999147, -31.15312499938548640, 96.81714838363319586 ) ) ;
#5935=CARTESIAN_POINT ( 'NONE',  ( -82.40000000000000568, -30.00000000000000355, 99.99999999999998579 ) ) ;
#5948=CARTESIAN_POINT ( 'NONE',  ( -83.90000000000000568, -31.22268749875867755, 102.5980762113533018 ) ) ;
#5949=CARTESIAN_POINT ( 'NONE',  ( -85.15643035624999868, -33.81562499938549138, 101.5914258081833879 ) ) ;
#5961=CARTESIAN_POINT ( 'NONE',  ( -85.15643035625001289, -32.42812499938548854, 98.40857419181659793 ) ) ;
#5972=CARTESIAN_POINT ( 'NONE',  ( -79.39999999999999147, -33.86250000000000426, 101.7320508075688537 ) ) ;
#5973=CARTESIAN_POINT ( 'NONE',  ( -79.39999999999999147, -31.10624999877097352, 101.7320508075688537 ) ) ;
#5984=CARTESIAN_POINT ( 'NONE',  ( -79.64356964375001269, -31.67812499938548143, 98.40857419181659793 ) ) ;
#5991=CARTESIAN_POINT ( 'NONE',  ( -80.90000000000000568, -30.75000000000000355, 102.5980762113533018 ) ) ;
#6005=CARTESIAN_POINT ( 'NONE',  ( -85.40000000000000568, -34.85624999877096997, 101.7320508075688821 ) ) ;
#6015=CARTESIAN_POINT ( 'NONE',  ( -79.39999999999999147, -31.10624999877097352, 101.7320508075688537 ) ) ;
#6017=CARTESIAN_POINT ( 'NONE',  ( -82.39999999999999147, -33.25856250001228887, 96.53589838486223584 ) ) ;
#6020=CARTESIAN_POINT ( 'NONE',  ( -83.77821517812500929, -31.11562499938548498, 97.61286128772489690 ) ) ;
#6021=CARTESIAN_POINT ( 'NONE',  ( -82.39999999999999147, -32.81250000000000000, 97.00000000000000000 ) ) ;
#6046=CARTESIAN_POINT ( 'NONE',  ( -79.39999999999999147, -31.11018749875868394, 101.7320508075688537 ) ) ;
#6047=CARTESIAN_POINT ( 'NONE',  ( -85.15643035624999868, -33.36562499938548854, 101.5914258081833879 ) ) ;
#6060=CARTESIAN_POINT ( 'NONE',  ( -79.64356964374998427, -32.57812499938548711, 98.40857419181659793 ) ) ;
#6070=CARTESIAN_POINT ( 'NONE',  ( -82.39999999999999147, -33.93750000000000000, 103.4641016151377499 ) ) ;
#6073=CARTESIAN_POINT ( 'NONE',  ( -82.39999999999999147, -32.53124999877096712, 103.4641016151377499 ) ) ;
#6085=CARTESIAN_POINT ( 'NONE',  ( -81.02178482187500208, -30.29062499938548569, 97.61286128772489690 ) ) ;
#6088=EDGE_LOOP ( 'NONE', ( #19059, #997 ) ) ;
#6091=CARTESIAN_POINT ( 'NONE',  ( -82.39999999999999147, -31.01249999999999929, 96.53589838486223584 ) ) ;
#6108=ORIENTED_EDGE ( 'NONE', *, *, #2563, .F. ) ;
#6113=CARTESIAN_POINT ( 'NONE',  ( -85.40000000000000568, -32.65856250001228744, 101.7320508075688679 ) ) ;
#6126=EDGE_CURVE ( 'NONE', #16779, #15015, #16013, .T. ) ;
#6127=CARTESIAN_POINT ( 'NONE',  ( -83.90000000000000568, -33.22500000000000142, 97.40192378864668399 ) ) ;
#6130=VERTEX_POINT ( 'NONE', #18753 ) ;
#6134=ADVANCED_FACE ( 'NONE', ( #877 ), #6840, .T. ) ;
#6139=CARTESIAN_POINT ( 'NONE',  ( -83.90000000000000568, -32.57268749875867542, 102.5980762113533018 ) ) ;
#6140=CARTESIAN_POINT ( 'NONE',  ( -81.02178482187500208, -33.70312499938548711, 102.3871387122750889 ) ) ;
#6156=CARTESIAN_POINT ( 'NONE',  ( -85.15643035625001289, -32.39062499938548711, 99.99999999999998579 ) ) ;
#6168=CARTESIAN_POINT ( 'NONE',  ( -85.40000000000000568, -30.84374999877096712, 99.99999999999998579 ) ) ;
#6169=CARTESIAN_POINT ( 'NONE',  ( -80.90000000000000568, -31.59374999877097423, 102.5980762113533018 ) ) ;
#6176=VERTEX_POINT ( 'NONE', #13255 ) ;
#6190=CARTESIAN_POINT ( 'NONE',  ( -82.39999999999999147, -31.46250000000000568, 96.53589838486223584 ) ) ;
#6204=CARTESIAN_POINT ( 'NONE',  ( -79.39999999999999147, -31.48124999877097352, 98.26794919243110371 ) ) ;
#6207=CARTESIAN_POINT ( 'NONE',  ( -85.15643035624999868, -31.56562499938548427, 101.5914258081833879 ) ) ;
#6211=CARTESIAN_POINT ( 'NONE',  ( -80.45107360500455229, -35.00092285196230080, 102.2869350179830121 ) ) ;
#6215=CARTESIAN_POINT ( 'NONE',  ( -85.40000000000000568, -34.94606250001229597, 99.99999999999998579 ) ) ;
#6217=CARTESIAN_POINT ( 'NONE',  ( -79.64356964374998427, -31.34062499938548640, 98.40857419181659793 ) ) ;
#6237=CARTESIAN_POINT ( 'NONE',  ( -85.40000000000000568, -31.74768749875867613, 99.99999999999998579 ) ) ;
#6243=CARTESIAN_POINT ( 'NONE',  ( -84.51155386534844638, -35.25364837475780888, 98.22820752270799005 ) ) ;
#6253=CARTESIAN_POINT ( 'NONE',  ( -84.51155153715826884, -35.14114847181267720, 98.22820474807231506 ) ) ;
#6257=CARTESIAN_POINT ( 'NONE',  ( -81.59615242270662350, -34.12634618820329990, 96.99999999999998579 ) ) ;
#6265=CARTESIAN_POINT ( 'NONE',  ( -85.40000000000000568, -34.46249999999999858, 101.7320508075688679 ) ) ;
#6266=CARTESIAN_POINT ( 'NONE',  ( -80.90000000000000568, -31.89374999877096784, 97.40192378864668399 ) ) ;
#6267=CARTESIAN_POINT ( 'NONE',  ( -85.40000000000000568, -30.19687499938548569, 99.99999999999998579 ) ) ;
#6268=CARTESIAN_POINT ( 'NONE',  ( -85.15643035625001289, -35.16562499938548569, 101.5914258081833879 ) ) ;
#6278=ORIENTED_EDGE ( 'NONE', *, *, #11010, .F. ) ;
#6283=ORIENTED_EDGE ( 'NONE', *, *, #10207, .F. ) ;
#6299=CARTESIAN_POINT ( 'NONE',  ( -79.64356964374999848, -30.47812499938548569, 99.99999999999998579 ) ) ;
#6304=CARTESIAN_POINT ( 'NONE',  ( -80.17521417250719651, -34.99920530278070885, 97.95730091510780824 ) ) ;
#6309=CARTESIAN_POINT ( 'NONE',  ( -85.15643035625001289, -30.74062499938548143, 98.40857419181659793 ) ) ;
#6310=CARTESIAN_POINT ( 'NONE',  ( -79.39999999999999147, -32.92500000000000426, 99.99999999999998579 ) ) ;
#6322=CARTESIAN_POINT ( 'NONE',  ( -83.20384757729335945, -33.24240381056766580, 96.99999999999998579 ) ) ;
#6333=CARTESIAN_POINT ( 'NONE',  ( -79.39999999999999147, -34.22268749875867400, 99.99999999999998579 ) ) ;
#6335=CARTESIAN_POINT ( 'NONE',  ( -79.64356964375001269, -34.94062499938549138, 98.40857419181659793 ) ) ;
#6348=EDGE_LOOP ( 'NONE', ( #2921, #3358, #8211, #16227 ) ) ;
#6353=CARTESIAN_POINT ( 'NONE',  ( -82.40000000000000568, -31.18124999877096926, 102.9999999999999858 ) ) ;
#6357=CARTESIAN_POINT ( 'NONE',  ( -83.90000000000000568, -34.87500000000000000, 102.5980762113533018 ) ) ;
#6358=CARTESIAN_POINT ( 'NONE',  ( -80.90000000000000568, -33.69374999877096855, 97.40192378864668399 ) ) ;
#6360=CARTESIAN_POINT ( 'NONE',  ( -80.90000000000000568, -30.75000000000000355, 102.5980762113533018 ) ) ;
#6390=EDGE_CURVE ( 'NONE', #9639, #6735, #3523, .T. ) ;
#6393=CARTESIAN_POINT ( 'NONE',  ( -79.64356964375001269, -32.31562499938548427, 101.5914258081833879 ) ) ;
#6398=CARTESIAN_POINT ( 'NONE',  ( -80.32324841350261124, -35.00093580010783256, 102.1718789886361094 ) ) ;
#6402=ADVANCED_FACE ( 'NONE', ( #6816 ), #11293, .T. ) ;
#6403=CARTESIAN_POINT ( 'NONE',  ( -85.15643035625001289, -32.54062499938548569, 98.40857419181659793 ) ) ;
#6415=DIRECTION ( 'NONE',  ( 0.000000000000000000, -1.000000000000000000, 0.000000000000000000 ) ) ;
#6424=CARTESIAN_POINT ( 'NONE',  ( -85.40000000000000568, -33.06018749875867258, 101.7320508075688679 ) ) ;
#6433=CARTESIAN_POINT ( 'NONE',  ( -85.40000000000000568, -30.00000000000000355, 99.99999999999998579 ) ) ;
#6436=ORIENTED_EDGE ( 'NONE', *, *, #5054, .T. ) ;
#6441=CARTESIAN_POINT ( 'NONE',  ( -82.39999999999999147, -34.07812499938548711, 103.1828516163667899 ) ) ;
#6447=CARTESIAN_POINT ( 'NONE',  ( -85.40000000000000568, -30.84374999877096712, 99.99999999999998579 ) ) ;
#6453=CARTESIAN_POINT ( 'NONE',  ( -79.39999999999999147, -32.83124999877097139, 98.26794919243110371 ) ) ;
#6454=CARTESIAN_POINT ( 'NONE',  ( -83.90000000000000568, -33.91874999877096997, 102.5980762113533018 ) ) ;
#6455=CARTESIAN_POINT ( 'NONE',  ( -79.39999999999999147, -30.61874999877096926, 99.99999999999998579 ) ) ;
#6470=EDGE_LOOP ( 'NONE', ( #10369, #9384, #18366, #12328 ) ) ;
#6474=CARTESIAN_POINT ( 'NONE',  ( -85.40000000000000568, -30.43124999877096926, 98.26794919243111792 ) ) ;
#6481=CARTESIAN_POINT ( 'NONE',  ( -82.40000000000000568, -30.00000000000000355, 99.99999999999998579 ) ) ;
#6490=CARTESIAN_POINT ( 'NONE',  ( -85.40000000000000568, -30.90000000000000213, 99.99999999999998579 ) ) ;
#6492=CARTESIAN_POINT ( 'NONE',  ( -79.64356964375001269, -31.79062499938548569, 98.40857419181659793 ) ) ;
#6504=EDGE_CURVE ( 'NONE', #19154, #4909, #6908, .T. ) ;
#6505=CARTESIAN_POINT ( 'NONE',  ( -83.77821517812500929, -31.22812499938548569, 97.61286128772489690 ) ) ;
#6523=CARTESIAN_POINT ( 'NONE',  ( -82.40000000000000568, -30.00000000000000355, 99.99999999999998579 ) ) ;
#6526=CARTESIAN_POINT ( 'NONE',  ( -85.40000000000000568, -34.93518749875867968, 98.26794919243111792 ) ) ;
#6530=PLANE ( 'NONE',  #15165 ) ;
#6539=CARTESIAN_POINT ( 'NONE',  ( -85.15643035624999868, -32.42812499938548854, 98.40857419181659793 ) ) ;
#6548=CARTESIAN_POINT ( 'NONE',  ( -83.20384757729337366, -31.20134618820330630, 102.9999999999999858 ) ) ;
#6551=CARTESIAN_POINT ( 'NONE',  ( -80.90000000000000568, -31.14374999877097139, 102.5980762113533018 ) ) ;
#6553=CARTESIAN_POINT ( 'NONE',  ( -85.40000000000000568, -33.58124999877097139, 98.26794919243111792 ) ) ;
#6562=CARTESIAN_POINT ( 'NONE',  ( -85.40000000000000568, -33.50624999877096855, 101.7320508075688821 ) ) ;
#6564=CARTESIAN_POINT ( 'NONE',  ( -82.40000000000000568, -30.00000000000000355, 99.99999999999998579 ) ) ;
#6565=EDGE_LOOP ( 'NONE', ( #18458, #18721, #3216, #13563, #17910, #5657, #13683, #12420, #1787, #8896, #8781, #18194, #8983, #11654, #1627, #15064, #12707, #15179, #15201, #11116, #149, #4590, #612, #4305, #2451 ) ) ;
#6573=CARTESIAN_POINT ( 'NONE',  ( -85.40000000000000568, -34.53356250001228744, 98.26794919243111792 ) ) ;
#6577=CARTESIAN_POINT ( 'NONE',  ( -79.39999999999999147, -33.37500000000000000, 99.99999999999998579 ) ) ;
#6587=CARTESIAN_POINT ( 'NONE',  ( -83.77821517812500929, -31.07812499938548711, 102.3871387122750889 ) ) ;
#6596=CARTESIAN_POINT ( 'NONE',  ( -79.64356964374998427, -31.41562499938548569, 101.5914258081833879 ) ) ;
#6609=DIRECTION ( 'NONE',  ( 0.000000000000000000, 0.000000000000000000, -1.000000000000000000 ) ) ;
#6612=( BOUNDED_SURFACE ( )  B_SPLINE_SURFACE ( 1, 2, ( 
 ( #12817, #14851, #23, #1475, #7433, #16708, #8890, #13390, #7622, #213, #12018, #4502, #3124, #11830, #316, #14755, #2938, #3032, #17990, #5973, #13575, #10648, #9081, #3221, #11923, #5880, #18090, #15143, #1760, #7717, #13677, #8799, #6169, #18181, #12120, #4699, #17797, #17894, #1387, #8991, #6266, #122, #4407, #16328, #10458, #13287, #10364, #12211, #16421, #10560, #4602, #16521, #14953, #19262, #1578, #7335, #7526, #6073, #13482, #4804, #15047, #16615, #1670, #9179, #10744, #11228, #16995, #4996, #12595, #3606, #16905, #4894, #789, #11125, #9567, #501, #9370, #13859, #15332, #1951, #3317, #3418, #7909, #2151, #14061, #6553, #18377, #15534, #6358, #14155, #9275, #16810, #3511, #12498, #6454, #8108, #5180, #696, #17093, #12406, #410, #18563, #9672, #15633, #2238, #8206, #15242, #6650, #12691, #3706, #10938, #9471, #6744, #18664, #1856, #18468, #18277, #5283, #7814, #13770, #12310, #10838, #15433, #2046, #8005, #13961, #604, #5088, #11031, #6936, #14247, #7213, #1070, #885, #12887 ),
 ( #8297, #10149, #3998, #16111, #18858, #13167, #15824, #18952, #5575, #11522, #8479, #8392, #3797, #3896, #14343, #10054, #7124, #12981, #1166, #9963, #2333, #17578, #14631, #17483, #4189, #4092, #5478, #16014, #2719, #17193, #2522, #14533, #9863, #6846, #11424, #981, #8678, #19043, #17385, #12791, #1266, #2617, #18760, #15917, #5379, #14436, #11327, #13077, #17292, #7027, #8578, #5666, #11609, #2433, #19138, #5755, #9766, #15728, #9059, #10625, #1451, #3005, #12091, #7404, #15024, #11807, #16590, #2914, #1362, #10431, #1555, #14726, #13459, #4572, #190, #11896, #13648, #8866, #1644, #10251, #15117, #14824, #16395, #6047, #5854, #13550, #1733, #7503, #13367, #1, #4287, #7691, #6140, #288, #17776, #5949, #17867, #3195, #11705, #17673, #16213, #16497, #4478, #4383, #18064, #95, #7597, #8963, #11994, #2819, #4675, #14930, #9154, #8776, #7306, #13263, #10340, #19237, #17962, #16304, #10530, #3100, #15506, #12474, #18537, #6335, #14125, #2215, #3582, #9541, #5153, #13935, #8178, #18442, #3289 ) ),
 .UNSPECIFIED., .F., .F., .F. ) 
 B_SPLINE_SURFACE_WITH_KNOTS ( ( 2, 2 ),
 ( 3, 2, 2, 2, 2, 2, 2, 2, 2, 2, 2, 2, 2, 2, 2, 2, 2, 2, 2, 2, 2, 2, 2, 2, 2, 2, 2, 2, 2, 2, 2, 2, 2, 2, 2, 2, 2, 2, 2, 2, 2, 2, 2, 2, 2, 2, 2, 2, 2, 2, 2, 2, 2, 2, 2, 2, 2, 2, 2, 2, 2, 2, 2, 2, 2, 2, 2, 3 ),
 ( 0.000000000000000000, 1.000000000000000000 ),
 ( 0.000000000000000000, 0.01388888888888888812, 0.02777777777777777624, 0.04166666666666666435, 0.05555555555555555247, 0.06944444444444444753, 0.08333333333333332871, 0.09722222222222222376, 0.1111111111111111049, 0.1250000000000000000, 0.1388888888888888951, 0.1527777777777777901, 0.1666666666666666574, 0.1805555555555555525, 0.1944444444444444475, 0.2083333333333333426, 0.2222222222222222099, 0.2361111111111111049, 0.2500000000000000000, 0.2638888888888888951, 0.2777777777777777901, 0.2916666666666666852, 0.3055555555555555802, 0.3194444444444444198, 0.3333333333333333148, 0.3472222222222222099, 0.3611111111111111049, 0.3750000000000000000, 0.3888888888888888951, 0.4027777777777777901, 0.4166666666666666852, 0.4305555555555555802, 0.4444444444444444198, 0.4583333333333333148, 0.4722222222222222099, 0.4861111111111111049, 0.5000000000000000000, 0.5138888888888888395, 0.5277777777777777901, 0.5416666666666666297, 0.5555555555555555802, 0.5694444444444444198, 0.5833333333333333703, 0.5972222222222222099, 0.6111111111111111605, 0.6250000000000000000, 0.6388888888888888395, 0.6527777777777777901, 0.6666666666666666297, 0.6805555555555555802, 0.6944444444444444198, 0.7083333333333333703, 0.7222222222222222099, 0.7361111111111111605, 0.7500000000000000000, 0.7638888888888888395, 0.7777777777777777901, 0.7916666666666666297, 0.8055555555555555802, 0.8194444444444444198, 0.8333333333333333703, 0.8472222222222222099, 0.8611111111111111605, 0.8750000000000000000, 0.8888888888888888395, 0.9027777777777777901, 0.9166666666666666297, 0.9258785144422092550 ),
 .UNSPECIFIED. ) 
 GEOMETRIC_REPRESENTATION_ITEM ( )  RATIONAL_B_SPLINE_SURFACE ( (
 ( 1.000000000000000000, 0.8660254037844387076, 1.000000000000000000, 0.8660254037844387076, 1.000000000000000000, 0.8660254037844387076, 1.000000000000000000, 0.8660254037844387076, 1.000000000000000000, 0.8660254037844387076, 1.000000000000000000, 0.8660254037844387076, 1.000000000000000000, 0.8660254037844387076, 1.000000000000000000, 0.8660254037844387076, 1.000000000000000000, 0.8660254037844387076, 1.000000000000000000, 0.8660254037844387076, 1.000000000000000000, 0.8660254037844387076, 1.000000000000000000, 0.8660254037844387076, 1.000000000000000000, 0.8660254037844387076, 1.000000000000000000, 0.8660254037844387076, 1.000000000000000000, 0.8660254037844387076, 1.000000000000000000, 0.8660254037844387076, 1.000000000000000000, 0.8660254037844387076, 1.000000000000000000, 0.8660254037844387076, 1.000000000000000000, 0.8660254037844387076, 1.000000000000000000, 0.8660254037844387076, 1.000000000000000000, 0.8660254037844387076, 1.000000000000000000, 0.8660254037844387076, 1.000000000000000000, 0.8660254037844387076, 1.000000000000000000, 0.8660254037844387076, 1.000000000000000000, 0.8660254037844387076, 1.000000000000000000, 0.8660254037844387076, 1.000000000000000000, 0.8660254037844387076, 1.000000000000000000, 0.8660254037844387076, 1.000000000000000000, 0.8660254037844387076, 1.000000000000000000, 0.8660254037844387076, 1.000000000000000000, 0.8660254037844387076, 1.000000000000000000, 0.8660254037844387076, 1.000000000000000000, 0.8660254037844387076, 1.000000000000000000, 0.8660254037844387076, 1.000000000000000000, 0.8660254037844387076, 1.000000000000000000, 0.8660254037844387076, 1.000000000000000000, 0.8660254037844387076, 1.000000000000000000, 0.8660254037844387076, 1.000000000000000000, 0.8660254037844387076, 1.000000000000000000, 0.8660254037844387076, 1.000000000000000000, 0.8660254037844387076, 1.000000000000000000, 0.8660254037844387076, 1.000000000000000000, 0.8660254037844387076, 1.000000000000000000, 0.8660254037844387076, 1.000000000000000000, 0.8660254037844387076, 1.000000000000000000, 0.8660254037844387076, 1.000000000000000000, 0.8660254037844387076, 1.000000000000000000, 0.8660254037844387076, 1.000000000000000000, 0.8660254037844387076, 1.000000000000000000, 0.8660254037844387076, 1.000000000000000000, 0.8660254037844387076, 1.000000000000000000, 0.8660254037844387076, 1.000000000000000000, 0.8660254037844387076, 1.000000000000000000, 0.8660254037844387076, 1.000000000000000000, 0.8660254037844387076, 1.000000000000000000, 0.8660254037844387076, 1.000000000000000000, 0.8660254037844387076, 1.000000000000000000, 0.8660254037844387076, 1.000000000000000000, 0.8660254037844387076, 1.000000000000000000, 0.8660254037844387076, 1.000000000000000000, 0.8660254037844387076, 1.000000000000000000, 0.8660254037844387076, 1.000000000000000000, 0.8660254037844387076, 1.000000000000000000, 0.8660254037844387076, 1.000000000000000000, 0.8660254037844387076, 1.000000000000000000, 0.8660254037844387076, 1.000000000000000000, 0.9111409417988175496, 0.9401539645359766606),
 ( 1.000000000000000000, 0.8660254037844387076, 1.000000000000000000, 0.8660254037844387076, 1.000000000000000000, 0.8660254037844387076, 1.000000000000000000, 0.8660254037844387076, 1.000000000000000000, 0.8660254037844387076, 1.000000000000000000, 0.8660254037844387076, 1.000000000000000000, 0.8660254037844387076, 1.000000000000000000, 0.8660254037844387076, 1.000000000000000000, 0.8660254037844387076, 1.000000000000000000, 0.8660254037844387076, 1.000000000000000000, 0.8660254037844387076, 1.000000000000000000, 0.8660254037844387076, 1.000000000000000000, 0.8660254037844387076, 1.000000000000000000, 0.8660254037844387076, 1.000000000000000000, 0.8660254037844387076, 1.000000000000000000, 0.8660254037844387076, 1.000000000000000000, 0.8660254037844387076, 1.000000000000000000, 0.8660254037844387076, 1.000000000000000000, 0.8660254037844387076, 1.000000000000000000, 0.8660254037844387076, 1.000000000000000000, 0.8660254037844387076, 1.000000000000000000, 0.8660254037844387076, 1.000000000000000000, 0.8660254037844387076, 1.000000000000000000, 0.8660254037844387076, 1.000000000000000000, 0.8660254037844387076, 1.000000000000000000, 0.8660254037844387076, 1.000000000000000000, 0.8660254037844387076, 1.000000000000000000, 0.8660254037844387076, 1.000000000000000000, 0.8660254037844387076, 1.000000000000000000, 0.8660254037844387076, 1.000000000000000000, 0.8660254037844387076, 1.000000000000000000, 0.8660254037844387076, 1.000000000000000000, 0.8660254037844387076, 1.000000000000000000, 0.8660254037844387076, 1.000000000000000000, 0.8660254037844387076, 1.000000000000000000, 0.8660254037844387076, 1.000000000000000000, 0.8660254037844387076, 1.000000000000000000, 0.8660254037844387076, 1.000000000000000000, 0.8660254037844387076, 1.000000000000000000, 0.8660254037844387076, 1.000000000000000000, 0.8660254037844387076, 1.000000000000000000, 0.8660254037844387076, 1.000000000000000000, 0.8660254037844387076, 1.000000000000000000, 0.8660254037844387076, 1.000000000000000000, 0.8660254037844387076, 1.000000000000000000, 0.8660254037844387076, 1.000000000000000000, 0.8660254037844387076, 1.000000000000000000, 0.8660254037844387076, 1.000000000000000000, 0.8660254037844387076, 1.000000000000000000, 0.8660254037844387076, 1.000000000000000000, 0.8660254037844387076, 1.000000000000000000, 0.8660254037844387076, 1.000000000000000000, 0.8660254037844387076, 1.000000000000000000, 0.8660254037844387076, 1.000000000000000000, 0.8660254037844387076, 1.000000000000000000, 0.8660254037844387076, 1.000000000000000000, 0.8660254037844387076, 1.000000000000000000, 0.8660254037844387076, 1.000000000000000000, 0.8660254037844387076, 1.000000000000000000, 0.8660254037844387076, 1.000000000000000000, 0.8660254037844387076, 1.000000000000000000, 0.8660254037844387076, 1.000000000000000000, 0.8660254037844387076, 1.000000000000000000, 0.8660254037844387076, 1.000000000000000000, 0.8660254037844387076, 1.000000000000000000, 0.8660254037844387076, 1.000000000000000000, 0.9111409417988175496, 0.9401539645359766606) ) ) 
 REPRESENTATION_ITEM ( '' )  SURFACE ( )  );
#6618=CARTESIAN_POINT ( 'NONE',  ( -80.90000000000000568, -35.04768749875867684, 97.40192378864668399 ) ) ;
#6635=CARTESIAN_POINT ( 'NONE',  ( -85.15643035624999868, -34.60312499938548569, 101.5914258081833879 ) ) ;
#6642=VERTEX_POINT ( 'NONE', #16747 ) ;
#6649=CARTESIAN_POINT ( 'NONE',  ( -80.90000000000000568, -30.99374999877096926, 97.40192378864668399 ) ) ;
#6650=CARTESIAN_POINT ( 'NONE',  ( -85.40000000000000568, -34.40624999877096712, 101.7320508075688679 ) ) ;
#6653=EDGE_CURVE ( 'NONE', #6130, #9315, #3410, .T. ) ;
#6660=CIRCLE ( 'NONE', #1039, 7.500000000000020428 ) ;
#6662=CARTESIAN_POINT ( 'NONE',  ( -82.40000000000000568, -50.00000000000000000, 99.99999999999998579 ) ) ;
#6676=CARTESIAN_POINT ( 'NONE',  ( -82.39999999999999147, -30.33750000000000213, 103.4641016151377499 ) ) ;
#6682=EDGE_LOOP ( 'NONE', ( #689, #9486, #1819, #16263 ) ) ;
#6685=CARTESIAN_POINT ( 'NONE',  ( -83.90000000000000568, -34.06874999877096855, 97.40192378864668399 ) ) ;
#6687=CARTESIAN_POINT ( 'NONE',  ( -85.15643035624999868, -34.79062499938548569, 98.40857419181659793 ) ) ;
#6696=CARTESIAN_POINT ( 'NONE',  ( -81.02178482187500208, -33.10312499938548569, 97.61286128772489690 ) ) ;
#6705=CARTESIAN_POINT ( 'NONE',  ( -85.40000000000000568, -33.05624999877097281, 101.7320508075688821 ) ) ;
#6708=CARTESIAN_POINT ( 'NONE',  ( -82.39999999999999147, -31.46249999999999858, 96.99999999999998579 ) ) ;
#6713=CARTESIAN_POINT ( 'NONE',  ( -81.59615242270662350, -32.96115380933864003, 103.0000000000000000 ) ) ;
#6715=CARTESIAN_POINT ( 'NONE',  ( -82.39999999999999147, -33.21018749875868536, 96.53589838486223584 ) ) ;
#6725=VERTEX_POINT ( 'NONE', #3841 ) ;
#6732=CARTESIAN_POINT ( 'NONE',  ( -85.15643035625001289, -33.29062499938547859, 99.99999999999998579 ) ) ;
#6735=VERTEX_POINT ( 'NONE', #9807 ) ;
#6738=ORIENTED_EDGE ( 'NONE', *, *, #2354, .T. ) ;
#6743=CARTESIAN_POINT ( 'NONE',  ( -85.40000000000000568, -33.13124999877096855, 98.26794919243111792 ) ) ;
#6744=CARTESIAN_POINT ( 'NONE',  ( -80.90000000000000568, -34.59374999877096712, 97.40192378864668399 ) ) ;
#6752=EDGE_CURVE ( 'NONE', #7637, #2550, #1418, .T. ) ;
#6761=CARTESIAN_POINT ( 'NONE',  ( -81.02178482187500208, -31.19062499938548427, 97.61286128772489690 ) ) ;
#6769=CYLINDRICAL_SURFACE ( 'NONE', #3309, 3.000000000000002665 ) ;
#6772=CARTESIAN_POINT ( 'NONE',  ( -79.39999999999999147, -34.30856250001229313, 101.7320508075688537 ) ) ;
#6779=ORIENTED_EDGE ( 'NONE', *, *, #14731, .T. ) ;
#6787=CARTESIAN_POINT ( 'NONE',  ( -79.64356964375001269, -33.59062499938548285, 98.40857419181659793 ) ) ;
#6791=DIRECTION ( 'NONE',  ( -0.000000000000000000, 1.000000000000000000, -0.000000000000000000 ) ) ;
#6799=CARTESIAN_POINT ( 'NONE',  ( -79.64356964374999848, -33.17812499938548854, 99.99999999999998579 ) ) ;
#6809=CARTESIAN_POINT ( 'NONE',  ( -83.90000000000000568, -32.32500000000000284, 97.40192378864668399 ) ) ;
#6816=FACE_OUTER_BOUND ( 'NONE', #12301, .T. ) ;
#6817=CARTESIAN_POINT ( 'NONE',  ( -85.40000000000000568, -30.00000000000000355, 99.99999999999998579 ) ) ;
#6836=CARTESIAN_POINT ( 'NONE',  ( -83.77821517812500929, -33.21562499938548285, 102.3871387122750889 ) ) ;
#6840=CYLINDRICAL_SURFACE ( 'NONE', #11291, 3.000000000000002665 ) ;
#6845=CARTESIAN_POINT ( 'NONE',  ( -83.90000000000000568, -32.11874999877097281, 102.5980762113533018 ) ) ;
#6846=CARTESIAN_POINT ( 'NONE',  ( -82.39999999999999147, -31.49062499938548854, 103.1828516163667899 ) ) ;
#6848=EDGE_CURVE ( 'NONE', #12516, #4275, #15870, .T. ) ;
#6852=VERTEX_POINT ( 'NONE', #930 ) ;
#6859=CARTESIAN_POINT ( 'NONE',  ( -83.77821517812500929, -30.96562499938548640, 102.3871387122750889 ) ) ;
#6869=CARTESIAN_POINT ( 'NONE',  ( -83.90000000000000568, -33.67106250001229739, 97.40192378864668399 ) ) ;
#6881=CARTESIAN_POINT ( 'NONE',  ( -83.77821517812500929, -33.47812499938548569, 97.61286128772489690 ) ) ;
#6885=CARTESIAN_POINT ( 'NONE',  ( -83.77821517812500929, -33.36562499938548854, 97.61286128772489690 ) ) ;
#6890=CARTESIAN_POINT ( 'NONE',  ( -85.15643035625001289, -33.36562499938548854, 101.5914258081833879 ) ) ;
#6901=CARTESIAN_POINT ( 'NONE',  ( -83.90000000000000568, -34.42500000000000426, 102.5980762113533018 ) ) ;
#6908=LINE ( 'NONE', #12857, #1317 ) ;
#6910=CARTESIAN_POINT ( 'NONE',  ( -85.40000000000000568, -30.89606250001229526, 99.99999999999998579 ) ) ;
#6912=DIRECTION ( 'NONE',  ( -0.000000000000000000, -1.000000000000000000, -0.000000000000000000 ) ) ;
#6914=FACE_OUTER_BOUND ( 'NONE', #11258, .T. ) ;
#6935=CARTESIAN_POINT ( 'NONE',  ( -80.90000000000000568, -35.04374999877096997, 97.40192378864668399 ) ) ;
#6936=CARTESIAN_POINT ( 'NONE',  ( -82.39999999999999147, -35.23124999877096997, 103.4641016151377499 ) ) ;
#6939=CARTESIAN_POINT ( 'NONE',  ( -82.40000000000000568, -30.00000000000000355, 103.0000000000000000 ) ) ;
#6948=CARTESIAN_POINT ( 'NONE',  ( -85.15643035625001289, -31.04062499938548569, 99.99999999999998579 ) ) ;
#6953=AXIS2_PLACEMENT_3D ( 'NONE', #7386, #14908, #1625 ) ;
#6959=CARTESIAN_POINT ( 'NONE',  ( -79.39999999999999147, -32.88750000000000284, 98.26794919243110371 ) ) ;
#6971=CARTESIAN_POINT ( 'NONE',  ( -81.02178482187500208, -32.65312499938548996, 97.61286128772489690 ) ) ;
#6974=VERTEX_POINT ( 'NONE', #10293 ) ;
#6975=CARTESIAN_POINT ( 'NONE',  ( -79.64356964375001269, -34.00312499938549138, 101.5914258081833879 ) ) ;
#6980=CARTESIAN_POINT ( 'NONE',  ( -79.64356964374998427, -34.04062499938549280, 98.40857419181659793 ) ) ;
#6992=CARTESIAN_POINT ( 'NONE',  ( -85.40000000000000568, -34.01250000000000284, 101.7320508075688679 ) ) ;
#6999=CARTESIAN_POINT ( 'NONE',  ( -79.39999999999999147, -30.18356250001229313, 98.26794919243110371 ) ) ;
#7002=CARTESIAN_POINT ( 'NONE',  ( -79.64356964375001269, -30.77812499938548285, 98.40857419181659793 ) ) ;
#7003=DIRECTION ( 'NONE',  ( -0.000000000000000000, -1.000000000000000000, -0.000000000000000000 ) ) ;
#7022=EDGE_CURVE ( 'NONE', #11515, #12396, #16882, .T. ) ;
#7026=CARTESIAN_POINT ( 'NONE',  ( -85.40000000000000568, -34.93124999877096570, 98.26794919243111792 ) ) ;
#7027=CARTESIAN_POINT ( 'NONE',  ( -85.15643035624999868, -32.09062499938548996, 98.40857419181659793 ) ) ;
#7038=CARTESIAN_POINT ( 'NONE',  ( -82.39999999999999147, -31.37812499938548427, 103.1828516163667899 ) ) ;
#7047=CARTESIAN_POINT ( 'NONE',  ( -80.90000000000000568, -31.65000000000000568, 102.5980762113533018 ) ) ;
#7052=CARTESIAN_POINT ( 'NONE',  ( -84.70833260042415702, -35.00006955123599539, 98.08383195543535749 ) ) ;
#7060=CARTESIAN_POINT ( 'NONE',  ( -82.39999999999999147, -33.96562499938548285, 96.81714838363319586 ) ) ;
#7061=DIRECTION ( 'NONE',  ( -0.6427825299241916035, 4.877271974511416535E-06, 0.7660487055014636448 ) ) ;
#7064=CARTESIAN_POINT ( 'NONE',  ( -79.64356964375001269, -33.92812499938548854, 98.40857419181659793 ) ) ;
#7067=APPLICATION_CONTEXT ( 'automotive_design' ) ;
#7071=CARTESIAN_POINT ( 'NONE',  ( -81.02178482187500208, -34.15312499938548285, 102.3871387122750889 ) ) ;
#7074=EDGE_CURVE ( 'NONE', #4275, #10919, #5427, .T. ) ;
#7084=CARTESIAN_POINT ( 'NONE',  ( -83.90000000000000568, -32.77499999999999858, 97.40192378864668399 ) ) ;
#7087=ORIENTED_EDGE ( 'NONE', *, *, #1328, .F. ) ;
#7093=FACE_OUTER_BOUND ( 'NONE', #14807, .T. ) ;
#7098=CARTESIAN_POINT ( 'NONE',  ( -83.20384757729335945, -33.69240381056766154, 96.99999999999998579 ) ) ;
#7100=EDGE_CURVE ( 'NONE', #1155, #2812, #1538, .T. ) ;
#7112=CARTESIAN_POINT ( 'NONE',  ( -79.64356964375001269, -34.90312499938548285, 101.5914258081833879 ) ) ;
#7123=CARTESIAN_POINT ( 'NONE',  ( -79.39999999999999147, -33.76874999877097139, 99.99999999999998579 ) ) ;
#7124=CARTESIAN_POINT ( 'NONE',  ( -81.02178482187500208, -30.85312499938548569, 97.61286128772489690 ) ) ;
#7133=EDGE_CURVE ( 'NONE', #6130, #14453, #3604, .T. ) ;
#7137=CARTESIAN_POINT ( 'NONE',  ( -83.77821517812500929, -31.41562499938548569, 102.3871387122750889 ) ) ;
#7148=CARTESIAN_POINT ( 'NONE',  ( -79.39999999999999147, -32.47500000000000142, 99.99999999999998579 ) ) ;
#7161=CARTESIAN_POINT ( 'NONE',  ( -84.51154815724953551, -35.25364861271051353, 98.22820072003833047 ) ) ;
#7165=CARTESIAN_POINT ( 'NONE',  ( -85.15643035624999868, -33.77812499938548285, 98.40857419181659793 ) ) ;
#7169=DIRECTION ( 'NONE',  ( -0.000000000000000000, -1.000000000000000000, -0.000000000000000000 ) ) ;
#7184=CARTESIAN_POINT ( 'NONE',  ( -85.40000000000000568, -30.41249999999999787, 101.7320508075688821 ) ) ;
#7190=CARTESIAN_POINT ( 'NONE',  ( -81.02178482187500208, -32.09062499938548285, 97.61286128772489690 ) ) ;
#7207=CARTESIAN_POINT ( 'NONE',  ( -79.39999999999999147, -30.18750000000000355, 98.26794919243110371 ) ) ;
#7212=CARTESIAN_POINT ( 'NONE',  ( -82.39999999999999147, -34.33124999877097139, 103.4641016151377499 ) ) ;
#7213=CARTESIAN_POINT ( 'NONE',  ( -85.40000000000000568, -35.30624999877096570, 101.7320508075688679 ) ) ;
#7225=CARTESIAN_POINT ( 'NONE',  ( -83.77821517812500929, -32.31562499938548427, 102.3871387122750889 ) ) ;
#7227=ORIENTED_EDGE ( 'NONE', *, *, #5561, .F. ) ;
#7238=CARTESIAN_POINT ( 'NONE',  ( -83.90000000000000568, -31.72500000000000142, 102.5980762113533018 ) ) ;
#7250=CARTESIAN_POINT ( 'NONE',  ( -85.15643035624999868, -30.55312499938548854, 101.5914258081833879 ) ) ;
#7251=CARTESIAN_POINT ( 'NONE',  ( -83.90000000000000568, -33.97500000000000853, 102.5980762113533018 ) ) ;
#7256=CARTESIAN_POINT ( 'NONE',  ( -85.40000000000000568, -31.76249999999999929, 101.7320508075688821 ) ) ;
#7257=CARTESIAN_POINT ( 'NONE',  ( -80.90000000000000568, -31.94999999999999929, 97.40192378864668399 ) ) ;
#7273=CARTESIAN_POINT ( 'NONE',  ( -80.90000000000000568, -34.80000000000000426, 102.5980762113533018 ) ) ;
#7281=CARTESIAN_POINT ( 'NONE',  ( -80.90000000000000568, -32.54606250001229739, 102.5980762113533018 ) ) ;
#7284=CARTESIAN_POINT ( 'NONE',  ( -81.02178482187500208, -32.69062499938548427, 102.3871387122750889 ) ) ;
#7299=ORIENTED_EDGE ( 'NONE', *, *, #4450, .F. ) ;
#7300=CARTESIAN_POINT ( 'NONE',  ( -80.90000000000000568, -30.30000000000000426, 102.5980762113533018 ) ) ;
#7305=CARTESIAN_POINT ( 'NONE',  ( -83.90000000000000568, -33.91874999877096997, 102.5980762113533018 ) ) ;
#7306=CARTESIAN_POINT ( 'NONE',  ( -79.64356964374999848, -34.52812499938548285, 99.99999999999998579 ) ) ;
#7309=LINE ( 'NONE', #13553, #1190 ) ;
#7314=EDGE_CURVE ( 'NONE', #12396, #16985, #8260, .T. ) ;
#7321=CARTESIAN_POINT ( 'NONE',  ( -85.15643035625001289, -32.80312499938548854, 101.5914258081833879 ) ) ;
#7333=CARTESIAN_POINT ( 'NONE',  ( -85.40000000000000568, -33.11250000000000426, 101.7320508075688679 ) ) ;
#7335=CARTESIAN_POINT ( 'NONE',  ( -79.39999999999999147, -32.45624999877097139, 101.7320508075688537 ) ) ;
#7337=CARTESIAN_POINT ( 'NONE',  ( -84.69814089128830403, -35.06584585096306483, 98.07164618293482761 ) ) ;
#7338=CYLINDRICAL_SURFACE ( 'NONE', #12732, 3.000000000000002665 ) ;
#7341=CARTESIAN_POINT ( 'NONE',  ( 0.000000000000000000, 0.000000000000000000, 0.000000000000000000 ) ) ;
#7347=CARTESIAN_POINT ( 'NONE',  ( -85.15643035625001289, -31.04062499938548569, 99.99999999999998579 ) ) ;
#7348=PLANE ( 'NONE',  #9734 ) ;
#7350=( BOUNDED_CURVE ( )  B_SPLINE_CURVE ( 2, ( #13314, #10102, #1312, #15872, #14779, #16058, #8623, #5709, #5521 ),
 .UNSPECIFIED., .F., .F. ) 
 B_SPLINE_CURVE_WITH_KNOTS ( ( 3, 2, 2, 2, 3 ),
 ( 0.4791666666666666297, 0.4861111111111111049, 0.5000000000000000000, 0.5138888888888888395, 0.5208333333333333703 ),
 .UNSPECIFIED. ) 
 CURVE ( )  GEOMETRIC_REPRESENTATION_ITEM ( )  RATIONAL_B_SPLINE_CURVE ( ( 0.9330127018922194093, 0.9330127018922190762, 1.000000000000000000, 0.8660254037844387076, 1.000000000000000000, 0.8660254037844387076, 1.000000000000000000, 0.9330127018922187432, 0.9330127018922192983 ) ) 
 REPRESENTATION_ITEM ( '' )  );
#7354=CARTESIAN_POINT ( 'NONE',  ( -80.90000000000000568, -30.60000000000000142, 97.40192378864668399 ) ) ;
#7369=FACE_OUTER_BOUND ( 'NONE', #2279, .T. ) ;
#7377=CARTESIAN_POINT ( 'NONE',  ( -79.39999999999999147, -32.88356250001229597, 98.26794919243110371 ) ) ;
#7380=CARTESIAN_POINT ( 'NONE',  ( -82.39999999999999147, -31.82812499938548356, 103.1828516163667899 ) ) ;
#7386=CARTESIAN_POINT ( 'NONE',  ( -82.40000000000000568, -30.00000000000000355, 99.99999999999998579 ) ) ;
#7388=ORIENTED_EDGE ( 'NONE', *, *, #6504, .T. ) ;
#7396=VECTOR ( 'NONE', #12095, 1000.000000000000000 ) ;
#7403=CARTESIAN_POINT ( 'NONE',  ( -85.40000000000000568, -32.64768749875867826, 99.99999999999998579 ) ) ;
#7404=CARTESIAN_POINT ( 'NONE',  ( -82.39999999999999147, -32.61562499938548854, 96.81714838363319586 ) ) ;
#7417=CARTESIAN_POINT ( 'NONE',  ( -81.02178482187500208, -33.59062499938548285, 102.3871387122750889 ) ) ;
#7422=CARTESIAN_POINT ( 'NONE',  ( -83.20384757729335945, -34.85759618943233562, 102.9999999999999716 ) ) ;
#7431=CARTESIAN_POINT ( 'NONE',  ( -79.39999999999999147, -33.37500000000000000, 99.99999999999998579 ) ) ;
#7433=CARTESIAN_POINT ( 'NONE',  ( -80.90000000000000568, -30.54374999877096997, 97.40192378864668399 ) ) ;
#7445=CARTESIAN_POINT ( 'NONE',  ( -83.77821517812500929, -30.66562499938548569, 97.61286128772489690 ) ) ;
#7446=CARTESIAN_POINT ( 'NONE',  ( -83.90000000000000568, -34.12500000000000000, 97.40192378864668399 ) ) ;
#7451=CARTESIAN_POINT ( 'NONE',  ( -85.40000000000000568, -30.48749999999999716, 98.26794919243111792 ) ) ;
#7473=CARTESIAN_POINT ( 'NONE',  ( -82.40000000000000568, -30.33749999999999858, 102.9999999999999858 ) ) ;
#7475=CARTESIAN_POINT ( 'NONE',  ( -79.39999999999999147, -32.43750000000000000, 98.26794919243110371 ) ) ;
#7476=CARTESIAN_POINT ( 'NONE',  ( -80.90000000000000568, -32.84606250001229455, 97.40192378864668399 ) ) ;
#7480=CARTESIAN_POINT ( 'NONE',  ( -79.64356964375001269, -31.67812499938548143, 98.40857419181659793 ) ) ;
#7481=CARTESIAN_POINT ( 'NONE',  ( -81.59615242270662350, -33.01740381056767148, 102.9999999999999858 ) ) ;
#7498=CARTESIAN_POINT ( 'NONE',  ( -82.40000000000000568, -30.11250000000000071, 96.99999999999998579 ) ) ;
#7502=CARTESIAN_POINT ( 'NONE',  ( -85.40000000000000568, -32.16018749875868110, 101.7320508075688679 ) ) ;
#7503=CARTESIAN_POINT ( 'NONE',  ( -82.39999999999999147, -33.51562499938548001, 96.81714838363319586 ) ) ;
#7509=ORIENTED_EDGE ( 'NONE', *, *, #7022, .T. ) ;
#7513=CARTESIAN_POINT ( 'NONE',  ( -83.77821517812500929, -34.26562499938548711, 97.61286128772489690 ) ) ;
#7525=CARTESIAN_POINT ( 'NONE',  ( -80.90000000000000568, -34.80000000000000426, 102.5980762113533018 ) ) ;
#7526=CARTESIAN_POINT ( 'NONE',  ( -80.90000000000000568, -32.49374999877097281, 102.5980762113533018 ) ) ;
#7527=LINE ( 'NONE', #6267, #18498 ) ;
#7537=CARTESIAN_POINT ( 'NONE',  ( -85.15643035624999868, -31.52812499938547930, 98.40857419181659793 ) ) ;
#7544=CARTESIAN_POINT ( 'NONE',  ( -82.39999999999999147, -31.23750000000000071, 103.4641016151377499 ) ) ;
#7551=EDGE_CURVE ( 'NONE', #6725, #9677, #17512, .T. ) ;
#7559=EDGE_CURVE ( 'NONE', #17250, #10662, #7566, .T. ) ;
#7566=CIRCLE ( 'NONE', #1329, 3.000000000000002665 ) ;
#7570=CARTESIAN_POINT ( 'NONE',  ( -85.40000000000000568, -32.24606250001229313, 99.99999999999998579 ) ) ;
#7596=CARTESIAN_POINT ( 'NONE',  ( -80.90000000000000568, -32.79768749875867684, 97.40192378864668399 ) ) ;
#7597=CARTESIAN_POINT ( 'NONE',  ( -83.77821517812500929, -34.22812499938549280, 102.3871387122750889 ) ) ;
#7598=CARTESIAN_POINT ( 'NONE',  ( -80.90000000000000568, -31.50000000000000000, 97.40192378864668399 ) ) ;
#7605=EDGE_LOOP ( 'NONE', ( #12809, #10134, #14970, #18887 ) ) ;
#7610=CARTESIAN_POINT ( 'NONE',  ( -85.15643035625001289, -33.32812499938548711, 98.40857419181659793 ) ) ;
#7611=ORIENTED_EDGE ( 'NONE', *, *, #5720, .T. ) ;
#7618=CARTESIAN_POINT ( 'NONE',  ( -84.51155153715826884, -35.14114847181267720, 98.22820474807231506 ) ) ;
#7621=CARTESIAN_POINT ( 'NONE',  ( -80.90000000000000568, -33.75000000000000000, 97.40192378864668399 ) ) ;
#7622=CARTESIAN_POINT ( 'NONE',  ( -80.90000000000000568, -30.69374999877097210, 102.5980762113533018 ) ) ;
#7624=CARTESIAN_POINT ( 'NONE',  ( -82.40000000000000568, -30.56250000000001066, 96.99999999999998579 ) ) ;
#7637=VERTEX_POINT ( 'NONE', #16522 ) ;
#7639=CARTESIAN_POINT ( 'NONE',  ( -79.39999999999999147, -31.61250000000000071, 101.7320508075688537 ) ) ;
#7644=DIRECTION ( 'NONE',  ( -0.000000000000000000, -1.000000000000000000, -0.000000000000000000 ) ) ;
#7656=CARTESIAN_POINT ( 'NONE',  ( -80.71939127259462055, -35.00048640298293634, 102.4907710001033507 ) ) ;
#7660=CARTESIAN_POINT ( 'NONE',  ( -82.39999999999999147, -33.48356250001229739, 103.4641016151377499 ) ) ;
#7661=EDGE_CURVE ( 'NONE', #10662, #15015, #11306, .T. ) ;
#7664=CARTESIAN_POINT ( 'NONE',  ( -79.64356964374999848, -32.27812499938548996, 99.99999999999998579 ) ) ;
#7672=VERTEX_POINT ( 'NONE', #14756 ) ;
#7675=EDGE_CURVE ( 'NONE', #15015, #17075, #7527, .T. ) ;
#7676=CARTESIAN_POINT ( 'NONE',  ( -85.40000000000000568, -33.11250000000000426, 101.7320508075688821 ) ) ;
#7684=LINE ( 'NONE', #9437, #14198 ) ;
#7689=CARTESIAN_POINT ( 'NONE',  ( -83.90000000000000568, -30.92268749875868039, 97.40192378864668399 ) ) ;
#7691=CARTESIAN_POINT ( 'NONE',  ( -79.64356964375001269, -33.66562499938549280, 101.5914258081833879 ) ) ;
#7696=B_SPLINE_CURVE_WITH_KNOTS ( 'NONE', 3,
 ( #450, #15377, #5033, #7853, #12058, #9316, #16561, #15280, #1704, #1994, #15180, #10597, #9214, #1895, #3163, #13612, #254, #7951, #10973, #13808, #7656, #6211, #6398, #12159, #18127, #4742, #10688, #16656, #1797, #3258, #7761, #13716, #357, #6304, #12254, #12352, #3838, #11071, #15767, #14291, #928, #18800 ),
 .UNSPECIFIED., .F., .F.,
 ( 4, 2, 2, 2, 2, 2, 2, 2, 2, 2, 2, 2, 2, 2, 2, 2, 2, 2, 2, 2, 4 ),
 ( 0.001272204158893248038, 0.06366052697277245487, 0.1260488497866516511, 0.1884371726005308612, 0.2508254954144100712, 0.3132138182282892536, 0.3444079796352281786, 0.3756021410421671036, 0.4379904638560474517, 0.5003787866699277442, 0.5315729480768661697, 0.5627671094838045951, 0.6251554322976795586, 0.6875437551115545221, 0.7187379165184906160, 0.7499320779254269320, 0.8123204007392985648, 0.8747087235531701976, 0.9059028849601048483, 0.9370970463670397210, 0.9994853691809091334 ),
 .UNSPECIFIED. ) ;
#7712=CARTESIAN_POINT ( 'NONE',  ( -82.40000000000000568, -30.00000000000000355, 99.99999999999998579 ) ) ;
#7716=CARTESIAN_POINT ( 'NONE',  ( -80.90000000000000568, -34.64999999999999858, 97.40192378864668399 ) ) ;
#7717=CARTESIAN_POINT ( 'NONE',  ( -79.39999999999999147, -31.48124999877097352, 98.26794919243110371 ) ) ;
#7719=MECHANICAL_DESIGN_GEOMETRIC_PRESENTATION_REPRESENTATION('',(#248),#2419);
#7757=CARTESIAN_POINT ( 'NONE',  ( -79.64356964374999848, -32.27812499938548996, 99.99999999999998579 ) ) ;
#7760=VERTEX_POINT ( 'NONE', #10649 ) ;
#7761=CARTESIAN_POINT ( 'NONE',  ( -79.46741390214279477, -35.00116912023187865, 99.34444296685866505 ) ) ;
#7767=CARTESIAN_POINT ( 'NONE',  ( -79.64356964374998427, -30.44062499938548783, 98.40857419181659793 ) ) ;
#7768=CARTESIAN_POINT ( 'NONE',  ( -80.90000000000000568, -32.85000000000000142, 97.40192378864668399 ) ) ;
#7788=CARTESIAN_POINT ( 'NONE',  ( -79.39999999999999147, -32.01018749875868252, 101.7320508075688537 ) ) ;
#7803=CARTESIAN_POINT ( 'NONE',  ( -81.02178482187500208, -34.79062499938548569, 97.61286128772489690 ) ) ;
#7812=CARTESIAN_POINT ( 'NONE',  ( -82.40000000000000568, -34.38749999999999574, 102.9999999999999858 ) ) ;
#7813=CARTESIAN_POINT ( 'NONE',  ( -82.39999999999999147, -34.61250000000000426, 96.53589838486223584 ) ) ;
#7814=CARTESIAN_POINT ( 'NONE',  ( -83.90000000000000568, -34.81874999877096855, 102.5980762113533018 ) ) ;
#7815=CARTESIAN_POINT ( 'NONE',  ( -80.90000000000000568, -30.54374999877096997, 97.40192378864668399 ) ) ;
#7816=ADVANCED_FACE ( 'NONE', ( #3222 ), #9180, .T. ) ;
#7833=ORIENTED_EDGE ( 'NONE', *, *, #10203, .T. ) ;
#7847=CARTESIAN_POINT ( 'NONE',  ( -83.20384757729335945, -30.99240381056766580, 96.99999999999998579 ) ) ;
#7849=CARTESIAN_POINT ( 'NONE',  ( -85.15643035625001289, -32.05312499938548854, 99.99999999999998579 ) ) ;
#7852=ORIENTED_EDGE ( 'NONE', *, *, #3186, .T. ) ;
#7853=CARTESIAN_POINT ( 'NONE',  ( -85.34334167081365763, -34.99814660107585951, 99.32349799501227494 ) ) ;
#7856=CARTESIAN_POINT ( 'NONE',  ( -79.39999999999999147, -34.63124999877096855, 98.26794919243110371 ) ) ;
#7861=CARTESIAN_POINT ( 'NONE',  ( -82.39999999999999147, -31.26562499938549067, 96.81714838363319586 ) ) ;
#7882=CARTESIAN_POINT ( 'NONE',  ( -80.90000000000000568, -33.24768749875867968, 97.40192378864668399 ) ) ;
#7884=DIRECTION ( 'NONE',  ( -0.000000000000000000, -1.000000000000000000, -0.000000000000000000 ) ) ;
#7897=CARTESIAN_POINT ( 'NONE',  ( -82.39999999999999147, -32.95312499938548711, 96.81714838363319586 ) ) ;
#7901=CARTESIAN_POINT ( 'NONE',  ( -82.40000000000000568, -30.73124999877097352, 102.9999999999999858 ) ) ;
#7903=VERTEX_POINT ( 'NONE', #13771 ) ;
#7907=CARTESIAN_POINT ( 'NONE',  ( -79.39999999999999147, -31.96874999877096712, 99.99999999999998579 ) ) ;
#7909=CARTESIAN_POINT ( 'NONE',  ( -83.90000000000000568, -33.46874999877096712, 102.5980762113533018 ) ) ;
#7910=CARTESIAN_POINT ( 'NONE',  ( -82.39999999999999147, -32.36250000000000426, 96.99999999999997158 ) ) ;
#7912=EDGE_CURVE ( 'NONE', #10919, #6974, #16257, .T. ) ;
#7917=FILL_AREA_STYLE_COLOUR ( '', #8347 ) ;
#7944=CARTESIAN_POINT ( 'NONE',  ( -82.39999999999999147, -30.78750000000000142, 102.9999999999999858 ) ) ;
#7946=CARTESIAN_POINT ( 'NONE',  ( -82.39999999999999147, -31.71562499938548640, 96.81714838363319586 ) ) ;
#7951=CARTESIAN_POINT ( 'NONE',  ( -81.62788447605926478, -34.99865355507268561, 102.9198516826838130 ) ) ;
#7955=CARTESIAN_POINT ( 'NONE',  ( -85.15643035625001289, -32.01562499938548001, 101.5914258081833879 ) ) ;
#7965=CARTESIAN_POINT ( 'NONE',  ( -82.39999999999999147, -32.98124999877096286, 102.9999999999999858 ) ) ;
#7976=CARTESIAN_POINT ( 'NONE',  ( -83.90000000000000568, -34.52268749875867826, 97.40192378864668399 ) ) ;
#7993=CARTESIAN_POINT ( 'NONE',  ( -81.02178482187500208, -32.69062499938548427, 102.3871387122750889 ) ) ;
#7994=VERTEX_POINT ( 'NONE', #15434 ) ;
#7997=CARTESIAN_POINT ( 'NONE',  ( -82.40000000000000568, -30.95624999877097139, 96.99999999999998579 ) ) ;
#8001=EDGE_CURVE ( 'NONE', #1272, #10334, #16140, .T. ) ;
#8004=CARTESIAN_POINT ( 'NONE',  ( -80.90000000000000568, -33.24374999877097281, 97.40192378864668399 ) ) ;
#8005=CARTESIAN_POINT ( 'NONE',  ( -80.90000000000000568, -35.04374999877096997, 97.40192378864668399 ) ) ;
#8014=CARTESIAN_POINT ( 'NONE',  ( -83.90000000000000568, -33.61874999877097281, 97.40192378864668399 ) ) ;
#8025=FACE_OUTER_BOUND ( 'NONE', #16887, .T. ) ;
#8028=CARTESIAN_POINT ( 'NONE',  ( -79.39999999999999147, -34.27106250001229171, 99.99999999999998579 ) ) ;
#8040=CARTESIAN_POINT ( 'NONE',  ( -85.40000000000000568, -33.99374999877097281, 99.99999999999998579 ) ) ;
#8042=CARTESIAN_POINT ( 'NONE',  ( -82.39999999999999147, -31.26562499938549067, 96.81714838363319586 ) ) ;
#8048=AXIS2_PLACEMENT_3D ( 'NONE', #9236, #13633, #467 ) ;
#8056=CARTESIAN_POINT ( 'NONE',  ( -79.64356964374999848, -31.37812499938548427, 99.99999999999998579 ) ) ;
#8064=EDGE_CURVE ( 'NONE', #12906, #13062, #917, .T. ) ;
#8068=CIRCLE ( 'NONE', #18998, 3.000000000000002665 ) ;
#8080=CARTESIAN_POINT ( 'NONE',  ( -85.40000000000000568, -33.99768749875867968, 99.99999999999998579 ) ) ;
#8086=CYLINDRICAL_SURFACE ( 'NONE', #9572, 3.000000000000002665 ) ;
#8096=CARTESIAN_POINT ( 'NONE',  ( -81.02178482187500208, -34.49062499938548854, 102.3871387122750889 ) ) ;
#8107=CARTESIAN_POINT ( 'NONE',  ( -80.90000000000000568, -31.89374999877096784, 97.40192378864668399 ) ) ;
#8108=CARTESIAN_POINT ( 'NONE',  ( -85.40000000000000568, -33.95624999877097139, 101.7320508075688679 ) ) ;
#8130=CARTESIAN_POINT ( 'NONE',  ( -80.90000000000000568, -30.15000000000000213, 97.40192378864668399 ) ) ;
#8142=CARTESIAN_POINT ( 'NONE',  ( -83.77821517812500929, -34.67812499938548854, 102.3871387122750889 ) ) ;
#8147=( BOUNDED_SURFACE ( )  B_SPLINE_SURFACE ( 1, 2, ( 
 ( #5259, #5357, #2593, #14505, #11587, #1050, #3873, #17552, #2404, #5548, #8368, #17360, #959, #3969, #12863, #9936, #2499, #7002, #2795, #1530, #17839, #16372, #2888, #5733, #10318, #19315, #6020, #5926, #5828, #4454, #11969, #10408, #8936, #14607, #11682, #3077, #17649, #11872, #4262, #11779, #14800, #7480, #14902, #9037, #17753, #7380, #15002, #14700, #1337, #67, #1238, #17937, #7190, #10221, #1427, #16187, #4358, #13436, #16278, #13340, #8844, #4549, #2980, #10505, #16472, #19113, #13139, #8748, #7284, #13238, #19211, #15768, #17524, #17330, #14571, #11365, #16153, #18708, #11561, #12926, #17432, #10098, #12835, #2765, #4136, #1208, #6885, #2659, #5425, #8431, #8620, #5329, #14476, #3939, #15957, #9906, #16054, #7165, #8526, #1106, #2562, #7064, #15869, #6975, #2475, #13115, #13023, #4043, #14384, #19086, #1023, #18897, #5705, #5517, #11465, #11656, #17234, #2376, #10002, #17618, #18995, #929, #12740, #4233, #5616, #10191, #18801, #8721, #14674, #1309, #11267, #3839, #9806, #8337, #14294, #17814, #18011 ),
 ( #4625, #10578, #233, #14973, #9197, #1687, #13212, #141, #15160, #4519, #16635, #17913, #4332, #7451, #3142, #18109, #7354, #9103, #13502, #12038, #5991, #10292, #13410, #1597, #13593, #9013, #2955, #6091, #16543, #4424, #10477, #10383, #15066, #7544, #16442, #8909, #19183, #40, #5900, #6190, #4721, #11846, #16252, #7639, #16345, #12140, #14871, #10665, #5798, #3239, #11942, #3051, #7257, #13310, #11750, #17721, #2861, #1402, #8818, #19284, #1499, #14774, #6809, #9822, #2393, #15978, #5242, #15885, #12943, #14494, #2679, #2490, #15784, #17448, #7084, #2582, #11577, #1226, #18724, #8355, #14309, #11191, #15691, #13040, #17348, #9727, #1038, #3860, #19011, #17154, #10019, #14400, #946, #8637, #8543, #11382, #4156, #3762, #5631, #10116, #5345, #16071, #2294, #8448, #14594, #17540, #18914, #6992, #12755, #11285, #12651, #18624, #1126, #8259, #14209, #5533, #846, #17253, #6901, #11482, #12850, #9924, #18821, #3958, #5444, #4059, #3067, #18031, #7273, #9029, #13427, #11957, #5916, #4251, #13327, #14889, #13518 ) ),
 .UNSPECIFIED., .F., .F., .F. ) 
 B_SPLINE_SURFACE_WITH_KNOTS ( ( 2, 2 ),
 ( 3, 2, 2, 2, 2, 2, 2, 2, 2, 2, 2, 2, 2, 2, 2, 2, 2, 2, 2, 2, 2, 2, 2, 2, 2, 2, 2, 2, 2, 2, 2, 2, 2, 2, 2, 2, 2, 2, 2, 2, 2, 2, 2, 2, 2, 2, 2, 2, 2, 2, 2, 2, 2, 2, 2, 2, 2, 2, 2, 2, 2, 2, 2, 2, 2, 2, 2, 2, 3 ),
 ( 0.000000000000000000, 1.000000000000000000 ),
 ( 0.000000000000000000, 0.01388888888888888812, 0.02777777777777777624, 0.04166666666666666435, 0.05555555555555555247, 0.06944444444444444753, 0.08333333333333332871, 0.09722222222222222376, 0.1111111111111111049, 0.1250000000000000000, 0.1388888888888888951, 0.1527777777777777901, 0.1666666666666666574, 0.1805555555555555525, 0.1944444444444444475, 0.2083333333333333426, 0.2222222222222222099, 0.2361111111111111049, 0.2500000000000000000, 0.2638888888888888951, 0.2777777777777777901, 0.2916666666666666852, 0.3055555555555555802, 0.3194444444444444198, 0.3333333333333333148, 0.3472222222222222099, 0.3611111111111111049, 0.3750000000000000000, 0.3888888888888888951, 0.4027777777777777901, 0.4166666666666666852, 0.4305555555555555802, 0.4444444444444444198, 0.4583333333333333148, 0.4722222222222222099, 0.4861111111111111049, 0.5000000000000000000, 0.5138888888888888395, 0.5277777777777777901, 0.5416666666666666297, 0.5555555555555555802, 0.5694444444444444198, 0.5833333333333333703, 0.5972222222222222099, 0.6111111111111111605, 0.6250000000000000000, 0.6388888888888888395, 0.6527777777777777901, 0.6666666666666666297, 0.6805555555555555802, 0.6944444444444444198, 0.7083333333333333703, 0.7222222222222222099, 0.7361111111111111605, 0.7500000000000000000, 0.7638888888888888395, 0.7777777777777777901, 0.7916666666666666297, 0.8055555555555555802, 0.8194444444444444198, 0.8333333333333333703, 0.8472222222222222099, 0.8611111111111111605, 0.8750000000000000000, 0.8888888888888888395, 0.9027777777777777901, 0.9166666666666666297, 0.9258785066912882389, 0.9351372917582011501 ),
 .UNSPECIFIED. ) 
 GEOMETRIC_REPRESENTATION_ITEM ( )  RATIONAL_B_SPLINE_SURFACE ( (
 ( 1.000000000000000000, 0.8660254037844387076, 1.000000000000000000, 0.8660254037844387076, 1.000000000000000000, 0.8660254037844387076, 1.000000000000000000, 0.8660254037844387076, 1.000000000000000000, 0.8660254037844387076, 1.000000000000000000, 0.8660254037844387076, 1.000000000000000000, 0.8660254037844387076, 1.000000000000000000, 0.8660254037844387076, 1.000000000000000000, 0.8660254037844387076, 1.000000000000000000, 0.8660254037844387076, 1.000000000000000000, 0.8660254037844387076, 1.000000000000000000, 0.8660254037844387076, 1.000000000000000000, 0.8660254037844387076, 1.000000000000000000, 0.8660254037844387076, 1.000000000000000000, 0.8660254037844387076, 1.000000000000000000, 0.8660254037844387076, 1.000000000000000000, 0.8660254037844387076, 1.000000000000000000, 0.8660254037844387076, 1.000000000000000000, 0.8660254037844387076, 1.000000000000000000, 0.8660254037844387076, 1.000000000000000000, 0.8660254037844387076, 1.000000000000000000, 0.8660254037844387076, 1.000000000000000000, 0.8660254037844387076, 1.000000000000000000, 0.8660254037844387076, 1.000000000000000000, 0.8660254037844387076, 1.000000000000000000, 0.8660254037844387076, 1.000000000000000000, 0.8660254037844387076, 1.000000000000000000, 0.8660254037844387076, 1.000000000000000000, 0.8660254037844387076, 1.000000000000000000, 0.8660254037844387076, 1.000000000000000000, 0.8660254037844387076, 1.000000000000000000, 0.8660254037844387076, 1.000000000000000000, 0.8660254037844387076, 1.000000000000000000, 0.8660254037844387076, 1.000000000000000000, 0.8660254037844387076, 1.000000000000000000, 0.8660254037844387076, 1.000000000000000000, 0.8660254037844387076, 1.000000000000000000, 0.8660254037844387076, 1.000000000000000000, 0.8660254037844387076, 1.000000000000000000, 0.8660254037844387076, 1.000000000000000000, 0.8660254037844387076, 1.000000000000000000, 0.8660254037844387076, 1.000000000000000000, 0.8660254037844387076, 1.000000000000000000, 0.8660254037844387076, 1.000000000000000000, 0.8660254037844387076, 1.000000000000000000, 0.8660254037844387076, 1.000000000000000000, 0.8660254037844387076, 1.000000000000000000, 0.8660254037844387076, 1.000000000000000000, 0.8660254037844387076, 1.000000000000000000, 0.8660254037844387076, 1.000000000000000000, 0.8660254037844387076, 1.000000000000000000, 0.8660254037844387076, 1.000000000000000000, 0.8660254037844387076, 1.000000000000000000, 0.8660254037844387076, 1.000000000000000000, 0.8660254037844387076, 1.000000000000000000, 0.8660254037844387076, 1.000000000000000000, 0.8660254037844387076, 1.000000000000000000, 0.8660254037844387076, 1.000000000000000000, 0.8660254037844387076, 1.000000000000000000, 0.8660254037844387076, 1.000000000000000000, 0.8660254037844387076, 1.000000000000000000, 0.8660254037844387076, 1.000000000000000000, 0.8660254037844387076, 1.000000000000000000, 0.8660254037844387076, 1.000000000000000000, 0.8660254037844387076, 1.000000000000000000, 0.8660254037844387076, 1.000000000000000000, 0.9111410165655264848, 0.9401539157124900736, 0.9401539157124900736, 0.9401539157124900736),
 ( 1.000000000000000000, 0.8660254037844387076, 1.000000000000000000, 0.8660254037844387076, 1.000000000000000000, 0.8660254037844387076, 1.000000000000000000, 0.8660254037844387076, 1.000000000000000000, 0.8660254037844387076, 1.000000000000000000, 0.8660254037844387076, 1.000000000000000000, 0.8660254037844387076, 1.000000000000000000, 0.8660254037844387076, 1.000000000000000000, 0.8660254037844387076, 1.000000000000000000, 0.8660254037844387076, 1.000000000000000000, 0.8660254037844387076, 1.000000000000000000, 0.8660254037844387076, 1.000000000000000000, 0.8660254037844387076, 1.000000000000000000, 0.8660254037844387076, 1.000000000000000000, 0.8660254037844387076, 1.000000000000000000, 0.8660254037844387076, 1.000000000000000000, 0.8660254037844387076, 1.000000000000000000, 0.8660254037844387076, 1.000000000000000000, 0.8660254037844387076, 1.000000000000000000, 0.8660254037844387076, 1.000000000000000000, 0.8660254037844387076, 1.000000000000000000, 0.8660254037844387076, 1.000000000000000000, 0.8660254037844387076, 1.000000000000000000, 0.8660254037844387076, 1.000000000000000000, 0.8660254037844387076, 1.000000000000000000, 0.8660254037844387076, 1.000000000000000000, 0.8660254037844387076, 1.000000000000000000, 0.8660254037844387076, 1.000000000000000000, 0.8660254037844387076, 1.000000000000000000, 0.8660254037844387076, 1.000000000000000000, 0.8660254037844387076, 1.000000000000000000, 0.8660254037844387076, 1.000000000000000000, 0.8660254037844387076, 1.000000000000000000, 0.8660254037844387076, 1.000000000000000000, 0.8660254037844387076, 1.000000000000000000, 0.8660254037844387076, 1.000000000000000000, 0.8660254037844387076, 1.000000000000000000, 0.8660254037844387076, 1.000000000000000000, 0.8660254037844387076, 1.000000000000000000, 0.8660254037844387076, 1.000000000000000000, 0.8660254037844387076, 1.000000000000000000, 0.8660254037844387076, 1.000000000000000000, 0.8660254037844387076, 1.000000000000000000, 0.8660254037844387076, 1.000000000000000000, 0.8660254037844387076, 1.000000000000000000, 0.8660254037844387076, 1.000000000000000000, 0.8660254037844387076, 1.000000000000000000, 0.8660254037844387076, 1.000000000000000000, 0.8660254037844387076, 1.000000000000000000, 0.8660254037844387076, 1.000000000000000000, 0.8660254037844387076, 1.000000000000000000, 0.8660254037844387076, 1.000000000000000000, 0.8660254037844387076, 1.000000000000000000, 0.8660254037844387076, 1.000000000000000000, 0.8660254037844387076, 1.000000000000000000, 0.8660254037844387076, 1.000000000000000000, 0.8660254037844387076, 1.000000000000000000, 0.8660254037844387076, 1.000000000000000000, 0.8660254037844387076, 1.000000000000000000, 0.8660254037844387076, 1.000000000000000000, 0.8660254037844387076, 1.000000000000000000, 0.8660254037844387076, 1.000000000000000000, 0.8660254037844387076, 1.000000000000000000, 0.8660254037844387076, 1.000000000000000000, 0.8660254037844387076, 1.000000000000000000, 0.8660254037844387076, 1.000000000000000000, 0.9111410165655264848, 0.9401539157124900736, 0.9401539157124900736, 0.9401539157124900736) ) ) 
 REPRESENTATION_ITEM ( '' )  SURFACE ( )  );
#8150=EDGE_CURVE ( 'NONE', #6852, #12897, #6660, .T. ) ;
#8152=CARTESIAN_POINT ( 'NONE',  ( -82.39999999999999147, -34.64062499938548711, 103.1828516163667899 ) ) ;
#8167=CARTESIAN_POINT ( 'NONE',  ( -83.20384757729335945, -31.44240381056766864, 97.00000000000000000 ) ) ;
#8173=CARTESIAN_POINT ( 'NONE',  ( -79.39999999999999147, -32.86874999877097281, 99.99999999999998579 ) ) ;
#8177=CARTESIAN_POINT ( 'NONE',  ( -83.90000000000000568, -34.37268749875867968, 102.5980762113533018 ) ) ;
#8178=CARTESIAN_POINT ( 'NONE',  ( -85.15643035625001289, -35.20312499938548711, 99.99999999999998579 ) ) ;
#8192=CARTESIAN_POINT ( 'NONE',  ( -79.64356964375001269, -34.37812499938548427, 98.40857419181659793 ) ) ;
#8203=CARTESIAN_POINT ( 'NONE',  ( -79.39999999999999147, -33.31874999877096855, 99.99999999999998579 ) ) ;
#8206=CARTESIAN_POINT ( 'NONE',  ( -82.39999999999999147, -34.33124999877097139, 103.4641016151377499 ) ) ;
#8211=ORIENTED_EDGE ( 'NONE', *, *, #14832, .T. ) ;
#8230=CARTESIAN_POINT ( 'NONE',  ( -82.39999999999999147, -34.15856250001229455, 96.53589838486223584 ) ) ;
#8234=CARTESIAN_POINT ( 'NONE',  ( -79.39999999999999147, -33.33749999999999858, 98.26794919243110371 ) ) ;
#8241=CARTESIAN_POINT ( 'NONE',  ( -79.64356964375001269, -34.94062499938549138, 98.40857419181659793 ) ) ;
#8250=CARTESIAN_POINT ( 'NONE',  ( -81.02178482187500208, -32.80312499938548854, 102.3871387122750889 ) ) ;
#8259=CARTESIAN_POINT ( 'NONE',  ( -79.39999999999999147, -34.23750000000000426, 98.26794919243110371 ) ) ;
#8260=( BOUNDED_CURVE ( )  B_SPLINE_CURVE ( 2, ( #5476, #17191, #8390, #4090, #5664, #8295, #9764, #17481, #15821 ),
 .UNSPECIFIED., .F., .F. ) 
 B_SPLINE_CURVE_WITH_KNOTS ( ( 3, 2, 2, 2, 3 ),
 ( 0.8125000000000000000, 0.8194444444444444198, 0.8333333333333333703, 0.8472222222222222099, 0.8541666666666665186 ),
 .UNSPECIFIED. ) 
 CURVE ( )  GEOMETRIC_REPRESENTATION_ITEM ( )  RATIONAL_B_SPLINE_CURVE ( ( 0.9330127018922194093, 0.9330127018922194093, 1.000000000000000000, 0.8660254037844387076, 1.000000000000000000, 0.8660254037844387076, 1.000000000000000000, 0.9330127018922209636, 0.9330127018922194093 ) ) 
 REPRESENTATION_ITEM ( '' )  );
#8266=EDGE_CURVE ( 'NONE', #11600, #7637, #13508, .T. ) ;
#8268=CARTESIAN_POINT ( 'NONE',  ( -82.39999999999999147, -30.78356250001229455, 103.4641016151377499 ) ) ;
#8269=CARTESIAN_POINT ( 'NONE',  ( -83.90000000000000568, -34.07268749875867542, 97.40192378864668399 ) ) ;
#8284=CARTESIAN_POINT ( 'NONE',  ( -83.77821517812500929, -32.91562499938547859, 97.61286128772489690 ) ) ;
#8295=CARTESIAN_POINT ( 'NONE',  ( -85.40000000000000568, -34.53750000000000142, 98.26794919243111792 ) ) ;
#8296=CARTESIAN_POINT ( 'NONE',  ( -79.39999999999999147, -31.93124999877096926, 98.26794919243110371 ) ) ;
#8297=CARTESIAN_POINT ( 'NONE',  ( -85.15643035625001289, -30.25312499938548783, 99.99999999999998579 ) ) ;
#8308=CARTESIAN_POINT ( 'NONE',  ( -84.70833260042415702, -35.00006955123599539, 98.08383195543535749 ) ) ;
#8312=CARTESIAN_POINT ( 'NONE',  ( -80.90000000000000568, -32.04374999877096997, 102.5980762113533018 ) ) ;
#8313=CARTESIAN_POINT ( 'NONE',  ( -82.40000000000000568, -50.00000000000000000, 92.49999999999997158 ) ) ;
#8315=( NAMED_UNIT ( * ) PLANE_ANGLE_UNIT ( ) SI_UNIT ( $, .RADIAN. ) );
#8319=CARTESIAN_POINT ( 'NONE',  ( -85.40000000000000568, -30.45000000000000284, 99.99999999999998579 ) ) ;
#8325=B_SPLINE_CURVE_WITH_KNOTS ( 'NONE', 3,
 ( #13102, #16331, #19072, #1389, #5690, #10174, #11641, #5883, #16138, #2846, #7337, #19265, #7052 ),
 .UNSPECIFIED., .F., .F.,
 ( 4, 3, 3, 3, 4 ),
 ( 1.387778780781445521E-17, 9.843749969274346115E-05, 0.0001968749993854869223, 0.0002955393327547696384, 0.0003942036661240663135 ),
 .UNSPECIFIED. ) ;
#8332=CARTESIAN_POINT ( 'NONE',  ( -79.64356964374999848, -34.97812499938548569, 99.99999999999998579 ) ) ;
#8337=CARTESIAN_POINT ( 'NONE',  ( -85.15643035624999868, -35.11426541925033007, 98.99674735228809652 ) ) ;
#8343=CARTESIAN_POINT ( 'NONE',  ( -85.15643035625001289, -32.99062499938548854, 98.40857419181659793 ) ) ;
#8347=COLOUR_RGB ( '',0.8941176470588234615, 0.8941176470588234615, 0.8941176470588234615 ) ;
#8355=CARTESIAN_POINT ( 'NONE',  ( -79.39999999999999147, -32.96250000000000568, 101.7320508075688537 ) ) ;
#8362=VECTOR ( 'NONE', #11154, 1000.000000000000000 ) ;
#8363=CARTESIAN_POINT ( 'NONE',  ( -79.39999999999999147, -32.41874999877096997, 99.99999999999998579 ) ) ;
#8365=CARTESIAN_POINT ( 'NONE',  ( -85.40000000000000568, -29.95276344769438737, 101.9998975609119469 ) ) ;
#8366=CARTESIAN_POINT ( 'NONE',  ( -80.90000000000000568, -34.80000000000000426, 102.5980762113533018 ) ) ;
#8368=CARTESIAN_POINT ( 'NONE',  ( -83.77821517812500929, -30.51562499938548711, 102.3871387122750889 ) ) ;
#8381=CARTESIAN_POINT ( 'NONE',  ( -85.15643035625001289, -35.09062499938548285, 99.99999999999998579 ) ) ;
#8390=CARTESIAN_POINT ( 'NONE',  ( -83.90000000000000568, -34.42500000000000426, 102.5980762113533018 ) ) ;
#8391=CARTESIAN_POINT ( 'NONE',  ( -85.40000000000000568, -33.58124999877097139, 98.26794919243111792 ) ) ;
#8392=CARTESIAN_POINT ( 'NONE',  ( -85.15643035624999868, -30.66562499938548569, 101.5914258081833879 ) ) ;
#8403=CARTESIAN_POINT ( 'NONE',  ( -82.39999999999999147, -35.23124999877096997, 103.4641016151377499 ) ) ;
#8404=CARTESIAN_POINT ( 'NONE',  ( -79.64356964374998427, -31.67812499938548143, 98.40857419181659793 ) ) ;
#8415=CARTESIAN_POINT ( 'NONE',  ( -80.90000000000000568, -32.55000000000000426, 102.5980762113533018 ) ) ;
#8417=ADVANCED_FACE ( 'NONE', ( #6914 ), #8147, .T. ) ;
#8420=CARTESIAN_POINT ( 'NONE',  ( -82.40000000000001990, -33.20624999877097849, 97.00000000000000000 ) ) ;
#8427=CARTESIAN_POINT ( 'NONE',  ( -85.15643035625001289, -34.30312499938548854, 99.99999999999998579 ) ) ;
#8431=CARTESIAN_POINT ( 'NONE',  ( -79.64356964375001269, -33.47812499938547859, 98.40857419181659793 ) ) ;
#8437=CARTESIAN_POINT ( 'NONE',  ( -81.02178482187500208, -34.90312499938548285, 97.61286128772489690 ) ) ;
#8448=CARTESIAN_POINT ( 'NONE',  ( -79.39999999999999147, -33.86250000000000426, 101.7320508075688537 ) ) ;
#8451=CARTESIAN_POINT ( 'NONE',  ( -83.20384757729335945, -31.25759618943233775, 102.9999999999999858 ) ) ;
#8454=CARTESIAN_POINT ( 'NONE',  ( -85.40000000000000568, -30.44606250001229242, 99.99999999999998579 ) ) ;
#8455=CARTESIAN_POINT ( 'NONE',  ( -79.39999999999999147, -34.76250000000000284, 101.7320508075688537 ) ) ;
#8458=CARTESIAN_POINT ( 'NONE',  ( -82.39999999999999147, -33.48750000000000426, 103.0000000000000000 ) ) ;
#8468=CARTESIAN_POINT ( 'NONE',  ( -85.15643035624999868, -35.11426555956768425, 98.99674139749697588 ) ) ;
#8478=CARTESIAN_POINT ( 'NONE',  ( -85.40000000000000568, -30.35438844644077605, 101.9998975609119469 ) ) ;
#8479=CARTESIAN_POINT ( 'NONE',  ( -83.77821517812500929, -30.62812499938548783, 102.3871387122750889 ) ) ;
#8493=CARTESIAN_POINT ( 'NONE',  ( -82.39999999999999147, -31.15312499938548640, 96.81714838363319586 ) ) ;
#8494=ORIENTED_EDGE ( 'NONE', *, *, #4260, .F. ) ;
#8505=CARTESIAN_POINT ( 'NONE',  ( -80.90000000000000568, -32.40000000000000568, 97.40192378864668399 ) ) ;
#8520=CARTESIAN_POINT ( 'NONE',  ( -79.64356964375001269, -33.66562499938549280, 101.5914258081833879 ) ) ;
#8526=CARTESIAN_POINT ( 'NONE',  ( -83.77821517812500929, -33.81562499938548427, 97.61286128772489690 ) ) ;
#8533=CARTESIAN_POINT ( 'NONE',  ( -79.64356964374998427, -33.66562499938548569, 101.5914258081833879 ) ) ;
#8543=CARTESIAN_POINT ( 'NONE',  ( -83.90000000000000568, -33.52499999999999858, 102.5980762113533018 ) ) ;
#8566=DIRECTION ( 'NONE',  ( -0.000000000000000000, -1.000000000000000000, -0.000000000000000000 ) ) ;
#8573=CARTESIAN_POINT ( 'NONE',  ( -82.40000000000000568, -32.08124999877097139, 102.9999999999999858 ) ) ;
#8577=CARTESIAN_POINT ( 'NONE',  ( -85.40000000000000568, -30.37603797259972893, 100.9999487804559664 ) ) ;
#8578=CARTESIAN_POINT ( 'NONE',  ( -83.77821517812500929, -32.12812499938548427, 97.61286128772489690 ) ) ;
#8591=CARTESIAN_POINT ( 'NONE',  ( -85.15643035625001289, -31.00312499938548427, 101.5914258081833879 ) ) ;
#8603=CARTESIAN_POINT ( 'NONE',  ( -85.40000000000000568, -31.31250000000000000, 101.7320508075688679 ) ) ;
#8616=CARTESIAN_POINT ( 'NONE',  ( -82.39999999999999147, -31.37812499938548427, 103.1828516163667899 ) ) ;
#8617=CARTESIAN_POINT ( 'NONE',  ( -82.40000000000000568, -33.93750000000000711, 102.9999999999999858 ) ) ;
#8619=ORIENTED_EDGE ( 'NONE', *, *, #13546, .T. ) ;
#8620=CARTESIAN_POINT ( 'NONE',  ( -79.64356964374999848, -33.51562499938548711, 99.99999999999998579 ) ) ;
#8623=CARTESIAN_POINT ( 'NONE',  ( -83.90000000000000568, -32.77499999999999858, 97.40192378864668399 ) ) ;
#8637=CARTESIAN_POINT ( 'NONE',  ( -82.39999999999999147, -33.48750000000000426, 103.4641016151377499 ) ) ;
#8644=CARTESIAN_POINT ( 'NONE',  ( -82.40000000000001990, -32.13750000000000284, 103.0000000000000000 ) ) ;
#8646=EDGE_CURVE ( 'NONE', #12516, #7903, #1950, .T. ) ;
#8649=CARTESIAN_POINT ( 'NONE',  ( -85.40000000000000568, -32.68124999877097281, 98.26794919243111792 ) ) ;
#8664=CARTESIAN_POINT ( 'NONE',  ( -85.15643035624999868, -34.67812499938548143, 98.40857419181659793 ) ) ;
#8670=ORIENTED_EDGE ( 'NONE', *, *, #13546, .F. ) ;
#8671=CARTESIAN_POINT ( 'NONE',  ( -83.90000000000000568, -32.11874999877097281, 102.5980762113533018 ) ) ;
#8677=CARTESIAN_POINT ( 'NONE',  ( -85.40000000000000568, -33.95624999877097139, 101.7320508075688679 ) ) ;
#8678=CARTESIAN_POINT ( 'NONE',  ( -85.15643035625001289, -31.60312499938548569, 99.99999999999998579 ) ) ;
#8685=EDGE_CURVE ( 'NONE', #2327, #16779, #5257, .T. ) ;
#8693=CARTESIAN_POINT ( 'NONE',  ( -85.15643035625001289, -30.14062499938548711, 99.99999999999998579 ) ) ;
#8695=ORIENTED_EDGE ( 'NONE', *, *, #13166, .T. ) ;
#8701=CARTESIAN_POINT ( 'NONE',  ( -83.20384757729335945, -31.65134618820330559, 102.9999999999999858 ) ) ;
#8705=CARTESIAN_POINT ( 'NONE',  ( -83.90000000000000568, -31.27500000000000568, 102.5980762113533018 ) ) ;
#8714=CARTESIAN_POINT ( 'NONE',  ( -79.64356964375001269, -30.40312499938548285, 101.5914258081833879 ) ) ;
#8715=CARTESIAN_POINT ( 'NONE',  ( -82.39999999999999147, -34.16250000000000142, 97.00000000000000000 ) ) ;
#8721=CARTESIAN_POINT ( 'NONE',  ( -79.64356964375001269, -34.90312499938548285, 101.5914258081833879 ) ) ;
#8727=CARTESIAN_POINT ( 'NONE',  ( -84.51155386534844638, -35.25364837475780888, 98.22820752270799005 ) ) ;
#8743=CARTESIAN_POINT ( 'NONE',  ( -85.40000000000000568, -32.28356250001229455, 98.26794919243111792 ) ) ;
#8748=CARTESIAN_POINT ( 'NONE',  ( -79.64356964375001269, -32.65312499938548285, 101.5914258081833879 ) ) ;
#8749=CARTESIAN_POINT ( 'NONE',  ( -82.40000000000001990, -32.53124999877097423, 103.0000000000000000 ) ) ;
#8769=CARTESIAN_POINT ( 'NONE',  ( -82.40000000000000568, -30.33749999999999858, 102.9999999999999858 ) ) ;
#8775=CARTESIAN_POINT ( 'NONE',  ( -85.40000000000000568, -33.54374999877096286, 99.99999999999998579 ) ) ;
#8776=CARTESIAN_POINT ( 'NONE',  ( -79.64356964375001269, -34.49062499938548854, 98.40857419181659793 ) ) ;
#8781=ORIENTED_EDGE ( 'NONE', *, *, #2671, .F. ) ;
#8785=CARTESIAN_POINT ( 'NONE',  ( -85.15643035625001289, -32.35312499938548569, 101.5914258081833879 ) ) ;
#8789=CARTESIAN_POINT ( 'NONE',  ( -80.90000000000000568, -34.29374999877096997, 102.5980762113533018 ) ) ;
#8798=CARTESIAN_POINT ( 'NONE',  ( -79.39999999999999147, -31.98750000000000071, 98.26794919243110371 ) ) ;
#8799=CARTESIAN_POINT ( 'NONE',  ( -79.39999999999999147, -31.55624999877096926, 101.7320508075688537 ) ) ;
#8809=AXIS2_PLACEMENT_3D ( 'NONE', #1224, #2781, #14398 ) ;
#8812=CARTESIAN_POINT ( 'NONE',  ( -85.15643035624999868, -35.16562499938547859, 101.5914258081833879 ) ) ;
#8815=VERTEX_POINT ( 'NONE', #14546 ) ;
#8818=CARTESIAN_POINT ( 'NONE',  ( -83.90000000000000568, -32.17500000000000426, 102.5980762113533018 ) ) ;
#8841=CARTESIAN_POINT ( 'NONE',  ( -83.90000000000000568, -32.62106250001229313, 102.5980762113533018 ) ) ;
#8844=CARTESIAN_POINT ( 'NONE',  ( -85.15643035625001289, -32.39062499938548711, 99.99999999999998579 ) ) ;
#8865=CARTESIAN_POINT ( 'NONE',  ( -85.40000000000000568, -30.81018749875867968, 101.7320508075688679 ) ) ;
#8866=CARTESIAN_POINT ( 'NONE',  ( -79.64356964375001269, -33.14062499938548711, 98.40857419181659793 ) ) ;
#8878=CARTESIAN_POINT ( 'NONE',  ( -79.64356964374999848, -34.41562499938548569, 99.99999999999998579 ) ) ;
#8889=CARTESIAN_POINT ( 'NONE',  ( -85.40000000000000568, -34.97364040220742964, 98.90809659374338025 ) ) ;
#8890=CARTESIAN_POINT ( 'NONE',  ( -79.39999999999999147, -30.61874999877096926, 99.99999999999998579 ) ) ;
#8896=ORIENTED_EDGE ( 'NONE', *, *, #54, .F. ) ;
#8902=CARTESIAN_POINT ( 'NONE',  ( -85.15643035625001289, -31.49062499938548498, 99.99999999999998579 ) ) ;
#8903=FACE_OUTER_BOUND ( 'NONE', #1222, .T. ) ;
#8907=CARTESIAN_POINT ( 'NONE',  ( -83.90000000000000568, -31.87500000000000000, 97.40192378864668399 ) ) ;
#8909=CARTESIAN_POINT ( 'NONE',  ( -85.40000000000000568, -31.31250000000000000, 101.7320508075688679 ) ) ;
#8925=FACE_OUTER_BOUND ( 'NONE', #6348, .T. ) ;
#8933=CARTESIAN_POINT ( 'NONE',  ( -82.39999999999999147, -32.80856250001228602, 96.53589838486223584 ) ) ;
#8936=CARTESIAN_POINT ( 'NONE',  ( -81.02178482187500208, -31.34062499938548996, 102.3871387122750889 ) ) ;
#8940=CARTESIAN_POINT ( 'NONE',  ( -82.40000000000001990, -33.26250000000000284, 97.00000000000000000 ) ) ;
#8960=CARTESIAN_POINT ( 'NONE',  ( -85.40000000000000568, -31.71018749875867115, 101.7320508075688679 ) ) ;
#8963=CARTESIAN_POINT ( 'NONE',  ( -85.15643035624999868, -34.26562499938548711, 101.5914258081833879 ) ) ;
#8964=CARTESIAN_POINT ( 'NONE',  ( -82.39999999999999147, -31.46249999999999858, 96.99999999999998579 ) ) ;
#8976=CARTESIAN_POINT ( 'NONE',  ( -79.64356964374998427, -33.92812499938548854, 98.40857419181659793 ) ) ;
#8978=ORIENTED_EDGE ( 'NONE', *, *, #7551, .T. ) ;
#8983=ORIENTED_EDGE ( 'NONE', *, *, #16654, .F. ) ;
#8990=CARTESIAN_POINT ( 'NONE',  ( -79.39999999999999147, -33.82500000000000284, 99.99999999999998579 ) ) ;
#8991=CARTESIAN_POINT ( 'NONE',  ( -82.39999999999999147, -31.85624999877097352, 96.53589838486223584 ) ) ;
#9006=CARTESIAN_POINT ( 'NONE',  ( -85.15643035624999868, -35.22676555956768141, 98.99674139749697588 ) ) ;
#9013=CARTESIAN_POINT ( 'NONE',  ( -85.40000000000000568, -30.93750000000000355, 98.26794919243111792 ) ) ;
#9025=CARTESIAN_POINT ( 'NONE',  ( -79.39999999999999147, -31.55624999877096926, 101.7320508075688537 ) ) ;
#9028=CARTESIAN_POINT ( 'NONE',  ( -83.90000000000000568, -34.81874999877096855, 102.5980762113533018 ) ) ;
#9029=CARTESIAN_POINT ( 'NONE',  ( -82.39999999999999147, -34.83749999999999858, 103.4641016151377499 ) ) ;
#9034=CARTESIAN_POINT ( 'NONE',  ( -80.90000000000000568, -32.09606250001229455, 102.5980762113533018 ) ) ;
#9037=CARTESIAN_POINT ( 'NONE',  ( -79.64356964375001269, -31.75312499938548427, 101.5914258081833879 ) ) ;
#9058=CARTESIAN_POINT ( 'NONE',  ( -82.39999999999999147, -32.98518749875867684, 103.4641016151377499 ) ) ;
#9059=CARTESIAN_POINT ( 'NONE',  ( -83.77821517812500929, -32.42812499938548854, 102.3871387122750889 ) ) ;
#9066=ORIENTED_EDGE ( 'NONE', *, *, #12261, .T. ) ;
#9071=CARTESIAN_POINT ( 'NONE',  ( -85.15643035625001289, -32.84062499938548285, 99.99999999999998579 ) ) ;
#9076=EDGE_LOOP ( 'NONE', ( #3622, #418, #10965, #6278 ) ) ;
#9080=CARTESIAN_POINT ( 'NONE',  ( -80.90000000000000568, -33.45000000000000284, 102.5980762113533018 ) ) ;
#9081=CARTESIAN_POINT ( 'NONE',  ( -83.90000000000000568, -31.21874999877097068, 102.5980762113533018 ) ) ;
#9095=CARTESIAN_POINT ( 'NONE',  ( -83.77821517812500929, -33.66562499938548569, 102.3871387122750889 ) ) ;
#9101=ORIENTED_EDGE ( 'NONE', *, *, #15736, .T. ) ;
#9103=CARTESIAN_POINT ( 'NONE',  ( -79.39999999999999147, -30.63750000000000284, 98.26794919243110371 ) ) ;
#9126=CARTESIAN_POINT ( 'NONE',  ( -81.59615242270663771, -31.16115380933863932, 103.0000000000000000 ) ) ;
#9127=CARTESIAN_POINT ( 'NONE',  ( -79.39999999999999147, -32.51250000000000284, 101.7320508075688537 ) ) ;
#9128=CARTESIAN_POINT ( 'NONE',  ( -79.39999999999999147, -32.95856250001229881, 101.7320508075688537 ) ) ;
#9130=CARTESIAN_POINT ( 'NONE',  ( -82.39999999999999147, -31.04062499938548569, 103.1828516163667899 ) ) ;
#9138=ORIENTED_EDGE ( 'NONE', *, *, #7100, .T. ) ;
#9148=EDGE_CURVE ( 'NONE', #13062, #4275, #3437, .T. ) ;
#9152=CARTESIAN_POINT ( 'NONE',  ( -82.39999999999999147, -31.18518749875867968, 103.4641016151377499 ) ) ;
#9154=CARTESIAN_POINT ( 'NONE',  ( -81.02178482187500208, -34.45312499938548711, 97.61286128772489690 ) ) ;
#9168=CARTESIAN_POINT ( 'NONE',  ( -82.39999999999999147, -33.40312499938548285, 96.81714838363319586 ) ) ;
#9178=CARTESIAN_POINT ( 'NONE',  ( -79.39999999999999147, -34.76250000000000284, 101.7320508075688537 ) ) ;
#9179=CARTESIAN_POINT ( 'NONE',  ( -82.39999999999999147, -32.75624999877096855, 96.53589838486223584 ) ) ;
#9180=CYLINDRICAL_SURFACE ( 'NONE', #5098, 3.000000000000002665 ) ;
#9197=CARTESIAN_POINT ( 'NONE',  ( -80.90000000000000568, -30.15000000000000213, 97.40192378864668399 ) ) ;
#9210=CARTESIAN_POINT ( 'NONE',  ( -81.02178482187500208, -31.90312499938548996, 102.3871387122750889 ) ) ;
#9214=CARTESIAN_POINT ( 'NONE',  ( -83.66537704785669405, -35.00036927961398447, 102.7253295689626782 ) ) ;
#9221=CARTESIAN_POINT ( 'NONE',  ( -82.39999999999999147, -32.16562499938548569, 96.81714838363319586 ) ) ;
#9233=CARTESIAN_POINT ( 'NONE',  ( -83.90000000000000568, -33.16874999877096286, 97.40192378864668399 ) ) ;
#9234=DIRECTION ( 'NONE',  ( -0.000000000000000000, -1.000000000000000000, -0.000000000000000000 ) ) ;
#9236=CARTESIAN_POINT ( 'NONE',  ( -82.40000000000000568, -30.00000000000000355, 99.99999999999998579 ) ) ;
#9237=ORIENTED_EDGE ( 'NONE', *, *, #9865, .T. ) ;
#9247=CARTESIAN_POINT ( 'NONE',  ( -80.90000000000000568, -30.99768749875867968, 97.40192378864668399 ) ) ;
#9263=CARTESIAN_POINT ( 'NONE',  ( -85.15643035625001289, -34.67812499938548143, 98.40857419181659793 ) ) ;
#9269=ORIENTED_EDGE ( 'NONE', *, *, #13688, .T. ) ;
#9271=CARTESIAN_POINT ( 'NONE',  ( -81.59615242270662350, -33.91740381056766296, 103.0000000000000000 ) ) ;
#9272=CARTESIAN_POINT ( 'NONE',  ( -83.90000000000000568, -33.52499999999999858, 102.5980762113533018 ) ) ;
#9275=CARTESIAN_POINT ( 'NONE',  ( -79.39999999999999147, -33.76874999877097139, 99.99999999999998579 ) ) ;
#9281=DIRECTION ( 'NONE',  ( -0.000000000000000000, -1.000000000000000000, -0.000000000000000000 ) ) ;
#9287=FACE_OUTER_BOUND ( 'NONE', #13472, .T. ) ;
#9293=EDGE_LOOP ( 'NONE', ( #16622, #2707, #13564, #17393 ) ) ;
#9299=CIRCLE ( 'NONE', #1807, 7.500000000000020428 ) ;
#9305=( BOUNDED_CURVE ( )  B_SPLINE_CURVE ( 2, ( #8458, #12956, #14321, #18927, #12864, #11496, #5642, #7098, #13055 ),
 .UNSPECIFIED., .F., .F. ) 
 B_SPLINE_CURVE_WITH_KNOTS ( ( 3, 2, 2, 2, 3 ),
 ( 0.6458333333333332593, 0.6527777777777777901, 0.6666666666666666297, 0.6805555555555555802, 0.6875000000000000000 ),
 .UNSPECIFIED. ) 
 CURVE ( )  GEOMETRIC_REPRESENTATION_ITEM ( )  RATIONAL_B_SPLINE_CURVE ( ( 0.9330127018922192983, 0.9330127018922187432, 1.000000000000000000, 0.8660254037844387076, 1.000000000000000000, 0.8660254037844387076, 1.000000000000000000, 0.9330127018922194093, 0.9330127018922194093 ) ) 
 REPRESENTATION_ITEM ( '' )  );
#9310=CARTESIAN_POINT ( 'NONE',  ( -85.40000000000000568, -30.86250000000000071, 101.7320508075688821 ) ) ;
#9312=CARTESIAN_POINT ( 'NONE',  ( -82.39999999999999147, -30.36562499938549209, 96.81714838363319586 ) ) ;
#9315=VERTEX_POINT ( 'NONE', #12517 ) ;
#9316=CARTESIAN_POINT ( 'NONE',  ( -85.40074734447198068, -35.00045574454757968, 100.3204239692404371 ) ) ;
#9320=CARTESIAN_POINT ( 'NONE',  ( -81.02178482187500208, -31.90312499938548996, 102.3871387122750889 ) ) ;
#9343=CARTESIAN_POINT ( 'NONE',  ( -83.90000000000000568, -33.62268749875867968, 97.40192378864668399 ) ) ;
#9355=B_SPLINE_CURVE_WITH_KNOTS ( 'NONE', 1,
 ( #2058, #4906 ),
 .UNSPECIFIED., .F., .F.,
 ( 2, 2 ),
 ( 0.000000000000000000, 1.000000000000000000 ),
 .UNSPECIFIED. ) ;
#9360=CARTESIAN_POINT ( 'NONE',  ( -83.77821517812500929, -34.71562499938548285, 97.61286128772489690 ) ) ;
#9361=ORIENTED_EDGE ( 'NONE', *, *, #10075, .F. ) ;
#9366=DIRECTION ( 'NONE',  ( 0.000000000000000000, 0.000000000000000000, -1.000000000000000000 ) ) ;
#9369=CARTESIAN_POINT ( 'NONE',  ( -85.40000000000000568, -32.64374999877097139, 99.99999999999998579 ) ) ;
#9370=CARTESIAN_POINT ( 'NONE',  ( -80.90000000000000568, -33.24374999877097281, 97.40192378864668399 ) ) ;
#9384=ORIENTED_EDGE ( 'NONE', *, *, #3608, .T. ) ;
#9399=DIRECTION ( 'NONE',  ( 0.000000000000000000, 0.000000000000000000, -1.000000000000000000 ) ) ;
#9408=CARTESIAN_POINT ( 'NONE',  ( -82.39999999999999147, -32.61562499938548854, 96.81714838363319586 ) ) ;
#9413=CARTESIAN_POINT ( 'NONE',  ( -79.39999999999999147, -34.66874999877096997, 99.99999999999998579 ) ) ;
#9415=AXIS2_PLACEMENT_3D ( 'NONE', #710, #3910, #14169 ) ;
#9418=CARTESIAN_POINT ( 'NONE',  ( -85.15643035625001289, -32.09062499938548996, 98.40857419181659793 ) ) ;
#9434=ORIENTED_EDGE ( 'NONE', *, *, #5054, .F. ) ;
#9436=CARTESIAN_POINT ( 'NONE',  ( -80.90000000000000568, -32.34374999877096712, 97.40192378864668399 ) ) ;
#9437=CARTESIAN_POINT ( 'NONE',  ( -82.40000000000000568, -30.00000000000000355, 96.99999999999998579 ) ) ;
#9440=CARTESIAN_POINT ( 'NONE',  ( -85.40000000000000568, -33.13518749875868252, 98.26794919243111792 ) ) ;
#9450=ORIENTED_EDGE ( 'NONE', *, *, #4839, .T. ) ;
#9456=CARTESIAN_POINT ( 'NONE',  ( -79.64356964375001269, -32.57812499938548001, 98.40857419181659793 ) ) ;
#9467=MANIFOLD_SOLID_BREP ( 'Thread1', #3526 ) ;
#9469=CARTESIAN_POINT ( 'NONE',  ( -79.39999999999999147, -32.06250000000000000, 101.7320508075688537 ) ) ;
#9470=CARTESIAN_POINT ( 'NONE',  ( -82.39999999999999147, -32.08124999877097139, 103.4641016151377499 ) ) ;
#9471=CARTESIAN_POINT ( 'NONE',  ( -82.39999999999999147, -34.55624999877096570, 96.53589838486223584 ) ) ;
#9486=ORIENTED_EDGE ( 'NONE', *, *, #13776, .T. ) ;
#9493=CARTESIAN_POINT ( 'NONE',  ( -85.40000000000000568, -34.08356250001229171, 98.26794919243111792 ) ) ;
#9496=EDGE_CURVE ( 'NONE', #16323, #12516, #18831, .T. ) ;
#9507=CARTESIAN_POINT ( 'NONE',  ( -79.64356964375001269, -31.34062499938548640, 98.40857419181659793 ) ) ;
#9519=CARTESIAN_POINT ( 'NONE',  ( -83.77821517812500929, -32.12812499938548427, 97.61286128772489690 ) ) ;
#9535=DIRECTION ( 'NONE',  ( -0.000000000000000000, -1.000000000000000000, -0.000000000000000000 ) ) ;
#9536=DIRECTION ( 'NONE',  ( 0.000000000000000000, 0.000000000000000000, -1.000000000000000000 ) ) ;
#9539=CARTESIAN_POINT ( 'NONE',  ( -85.40000000000000568, -34.48518749875868394, 98.26794919243111792 ) ) ;
#9541=CARTESIAN_POINT ( 'NONE',  ( -82.39999999999999147, -35.09062499938548285, 103.1828516163667899 ) ) ;
#9542=CARTESIAN_POINT ( 'NONE',  ( -82.40000000000000568, -35.00000000000000000, 99.99999999999998579 ) ) ;
#9543=CARTESIAN_POINT ( 'NONE',  ( -85.27821517812500929, -30.07031249969274356, 99.99999999999998579 ) ) ;
#9555=CARTESIAN_POINT ( 'NONE',  ( -79.64356964374999848, -34.41562499938548569, 99.99999999999998579 ) ) ;
#9557=ORIENTED_EDGE ( 'NONE', *, *, #6752, .T. ) ;
#9566=CARTESIAN_POINT ( 'NONE',  ( -83.90000000000000568, -33.16874999877096286, 97.40192378864668399 ) ) ;
#9567=CARTESIAN_POINT ( 'NONE',  ( -83.90000000000000568, -33.16874999877096286, 97.40192378864668399 ) ) ;
#9568=CARTESIAN_POINT ( 'NONE',  ( -83.20384757729337366, -32.34240381056766722, 97.00000000000000000 ) ) ;
#9572=AXIS2_PLACEMENT_3D ( 'NONE', #3686, #15412, #17173 ) ;
#9585=CARTESIAN_POINT ( 'NONE',  ( -80.90000000000000568, -31.89374999877096784, 97.40192378864668399 ) ) ;
#9595=CARTESIAN_POINT ( 'NONE',  ( -84.69814161231455785, -34.99658579608068720, 98.07164704222793716 ) ) ;
#9596=DIRECTION ( 'NONE',  ( 0.000000000000000000, 0.000000000000000000, -1.000000000000000000 ) ) ;
#9610=CARTESIAN_POINT ( 'NONE',  ( -81.02178482187500208, -30.55312499938548854, 102.3871387122750889 ) ) ;
#9623=CARTESIAN_POINT ( 'NONE',  ( -83.77821517812500929, -34.22812499938549280, 102.3871387122750889 ) ) ;
#9630=VERTEX_POINT ( 'NONE', #3119 ) ;
#9632=CARTESIAN_POINT ( 'NONE',  ( -82.40000000000000568, -30.56250000000001066, 96.99999999999998579 ) ) ;
#9633=AXIS2_PLACEMENT_3D ( 'NONE', #10412, #73, #1535 ) ;
#9637=EDGE_CURVE ( 'NONE', #9315, #2507, #14815, .T. ) ;
#9638=CARTESIAN_POINT ( 'NONE',  ( -85.40000000000000568, -31.38749999999999929, 98.26794919243111792 ) ) ;
#9639=VERTEX_POINT ( 'NONE', #10643 ) ;
#9642=CARTESIAN_POINT ( 'NONE',  ( -82.40000000000001990, -32.53124999877097423, 103.0000000000000000 ) ) ;
#9644=CARTESIAN_POINT ( 'NONE',  ( -79.39999999999999147, -32.90624999877096712, 101.7320508075688537 ) ) ;
#9646=CARTESIAN_POINT ( 'NONE',  ( -80.90000000000000568, -34.59768749875867400, 97.40192378864668399 ) ) ;
#9647=EDGE_CURVE ( 'NONE', #9630, #7994, #11387, .T. ) ;
#9660=CARTESIAN_POINT ( 'NONE',  ( -85.15643035624999868, -33.70312499938548711, 101.5914258081833879 ) ) ;
#9665=DIRECTION ( 'NONE',  ( 0.000000000000000000, 0.000000000000000000, -1.000000000000000000 ) ) ;
#9670=CARTESIAN_POINT ( 'NONE',  ( -79.39999999999999147, -31.98750000000000071, 98.26794919243110371 ) ) ;
#9671=CARTESIAN_POINT ( 'NONE',  ( -82.39999999999999147, -32.98124999877096997, 103.4641016151377499 ) ) ;
#9672=CARTESIAN_POINT ( 'NONE',  ( -79.39999999999999147, -34.21874999877096712, 99.99999999999998579 ) ) ;
#9677=VERTEX_POINT ( 'NONE', #7618 ) ;
#9682=DIRECTION ( 'NONE',  ( 0.000000000000000000, -0.000000000000000000, 1.000000000000000000 ) ) ;
#9688=ORIENTED_EDGE ( 'NONE', *, *, #18429, .F. ) ;
#9689=( NAMED_UNIT ( * ) SI_UNIT ( $, .STERADIAN. ) SOLID_ANGLE_UNIT ( ) );
#9693=CARTESIAN_POINT ( 'NONE',  ( -85.40000000000000568, -30.48749999999999716, 98.26794919243111792 ) ) ;
#9699=CARTESIAN_POINT ( 'NONE',  ( -79.39999999999999147, -31.12500000000000355, 99.99999999999998579 ) ) ;
#9707=CARTESIAN_POINT ( 'NONE',  ( -83.77821517812500929, -34.82812499938548711, 97.61286128772489690 ) ) ;
#9716=CARTESIAN_POINT ( 'NONE',  ( -82.39999999999999147, -33.06562499938548427, 96.81714838363319586 ) ) ;
#9723=ADVANCED_FACE ( 'NONE', ( #18085 ), #15138, .T. ) ;
#9727=CARTESIAN_POINT ( 'NONE',  ( -85.40000000000000568, -33.18750000000000000, 98.26794919243111792 ) ) ;
#9734=AXIS2_PLACEMENT_3D ( 'NONE', #13302, #7061, #18992 ) ;
#9735=CARTESIAN_POINT ( 'NONE',  ( -80.90000000000000568, -32.49374999877097281, 102.5980762113533018 ) ) ;
#9737=CARTESIAN_POINT ( 'NONE',  ( -79.39999999999999147, -30.67106250001229029, 99.99999999999998579 ) ) ;
#9738=CARTESIAN_POINT ( 'NONE',  ( -85.40000000000000568, -34.86018749875868394, 101.7320508075688679 ) ) ;
#9752=CARTESIAN_POINT ( 'NONE',  ( -81.02178482187500208, -32.99062499938548854, 97.61286128772489690 ) ) ;
#9764=CARTESIAN_POINT ( 'NONE',  ( -83.90000000000000568, -34.57500000000000284, 97.40192378864668399 ) ) ;
#9765=CARTESIAN_POINT ( 'NONE',  ( -79.39999999999999147, -32.00624999877096855, 101.7320508075688537 ) ) ;
#9766=CARTESIAN_POINT ( 'NONE',  ( -81.02178482187500208, -32.35312499938548569, 102.3871387122750889 ) ) ;
#9778=CARTESIAN_POINT ( 'NONE',  ( -83.04637810842696410, -35.00000000000000711, 97.04408774215416145 ) ) ;
#9789=CARTESIAN_POINT ( 'NONE',  ( -85.40000000000000568, -30.00000000000000355, 99.99999999999998579 ) ) ;
#9802=CARTESIAN_POINT ( 'NONE',  ( -81.02178482187500208, -33.55312499938548854, 97.61286128772489690 ) ) ;
#9806=CARTESIAN_POINT ( 'NONE',  ( -85.15643035625001289, -35.09062499938548285, 99.99999999999998579 ) ) ;
#9807=CARTESIAN_POINT ( 'NONE',  ( -82.40000000000001990, -32.53124999877097423, 103.0000000000000000 ) ) ;
#9812=CARTESIAN_POINT ( 'NONE',  ( -79.64356964374998427, -32.69062499938548427, 98.40857419181659793 ) ) ;
#9822=CARTESIAN_POINT ( 'NONE',  ( -82.39999999999999147, -32.36250000000000426, 96.53589838486223584 ) ) ;
#9831=CARTESIAN_POINT ( 'NONE',  ( -80.90000000000000568, -30.14606250001229171, 97.40192378864668399 ) ) ;
#9843=ORIENTED_EDGE ( 'NONE', *, *, #7314, .T. ) ;
#9854=EDGE_CURVE ( 'NONE', #7903, #9639, #716, .T. ) ;
#9862=CARTESIAN_POINT ( 'NONE',  ( -79.39999999999999147, -34.21874999877096712, 99.99999999999998579 ) ) ;
#9863=CARTESIAN_POINT ( 'NONE',  ( -81.02178482187500208, -31.45312499938549067, 102.3871387122750889 ) ) ;
#9864=LINE ( 'NONE', #6939, #11178 ) ;
#9865=EDGE_CURVE ( 'NONE', #14886, #7672, #11933, .T. ) ;
#9876=CARTESIAN_POINT ( 'NONE',  ( -85.15643035625001289, -31.97812499938548925, 98.40857419181659793 ) ) ;
#9888=CARTESIAN_POINT ( 'NONE',  ( -83.90000000000000568, -34.42106250001229739, 102.5980762113533018 ) ) ;
#9896=VECTOR ( 'NONE', #5697, 1000.000000000000000 ) ;
#9899=CARTESIAN_POINT ( 'NONE',  ( -82.40000000000000568, -33.43124999877096570, 102.9999999999999858 ) ) ;
#9901=CARTESIAN_POINT ( 'NONE',  ( -79.64356964374999848, -34.07812499938548711, 99.99999999999998579 ) ) ;
#9904=ORIENTED_EDGE ( 'NONE', *, *, #3186, .F. ) ;
#9906=CARTESIAN_POINT ( 'NONE',  ( -85.15643035624999868, -33.70312499938548711, 101.5914258081833879 ) ) ;
#9912=CARTESIAN_POINT ( 'NONE',  ( -79.64356964374999848, -34.52812499938548285, 99.99999999999998579 ) ) ;
#9915=( GEOMETRIC_REPRESENTATION_CONTEXT ( 3 ) GLOBAL_UNCERTAINTY_ASSIGNED_CONTEXT ( ( #12511 ) ) GLOBAL_UNIT_ASSIGNED_CONTEXT ( ( #15251, #16818, #4710 ) ) REPRESENTATION_CONTEXT ( 'NONE', 'WORKASPACE' ) );
#9924=CARTESIAN_POINT ( 'NONE',  ( -85.40000000000000568, -34.53750000000000142, 98.26794919243111792 ) ) ;
#9932=CARTESIAN_POINT ( 'NONE',  ( -83.90000000000000568, -30.82106250001229242, 102.5980762113533018 ) ) ;
#9936=CARTESIAN_POINT ( 'NONE',  ( -82.39999999999999147, -30.70312499938548711, 96.81714838363319586 ) ) ;
#9943=( BOUNDED_CURVE ( )  B_SPLINE_CURVE ( 2, ( #11492, #3871, #10028, #11585, #14503, #8455, #8366, #11680, #2689 ),
 .UNSPECIFIED., .F., .F. ) 
 B_SPLINE_CURVE_WITH_KNOTS ( ( 3, 2, 2, 2, 3 ),
 ( 0.8541666666666665186, 0.8611111111111111605, 0.8750000000000000000, 0.8888888888888888395, 0.8958333333333333703 ),
 .UNSPECIFIED. ) 
 CURVE ( )  GEOMETRIC_REPRESENTATION_ITEM ( )  RATIONAL_B_SPLINE_CURVE ( ( 0.9330127018922194093, 0.9330127018922177440, 1.000000000000000000, 0.8660254037844387076, 1.000000000000000000, 0.8660254037844387076, 1.000000000000000000, 0.9330127018922187432, 0.9330127018922192983 ) ) 
 REPRESENTATION_ITEM ( '' )  );
#9951=CARTESIAN_POINT ( 'NONE',  ( -82.40000000000000568, -30.00000000000000355, 99.99999999999998579 ) ) ;
#9962=CARTESIAN_POINT ( 'NONE',  ( -82.39999999999999147, -34.55624999877096570, 96.53589838486223584 ) ) ;
#9963=CARTESIAN_POINT ( 'NONE',  ( -79.64356964375001269, -30.96562499938548640, 101.5914258081833879 ) ) ;
#9976=CARTESIAN_POINT ( 'NONE',  ( -85.15643035625001289, -30.59062499938548285, 99.99999999999998579 ) ) ;
#9979=CARTESIAN_POINT ( 'NONE',  ( -79.39999999999999147, -31.96874999877096712, 99.99999999999998579 ) ) ;
#9981=ORIENTED_EDGE ( 'NONE', *, *, #4839, .F. ) ;
#9986=CARTESIAN_POINT ( 'NONE',  ( -85.40000000000000568, -31.35000000000000142, 99.99999999999998579 ) ) ;
#9998=CARTESIAN_POINT ( 'NONE',  ( -79.64356964374999848, -33.17812499938548854, 99.99999999999998579 ) ) ;
#10002=CARTESIAN_POINT ( 'NONE',  ( -83.77821517812500929, -34.56562499938548427, 102.3871387122750889 ) ) ;
#10007=CARTESIAN_POINT ( 'NONE',  ( -82.39999999999999147, -34.16250000000000142, 97.00000000000000000 ) ) ;
#10008=CARTESIAN_POINT ( 'NONE',  ( -79.64356964374998427, -32.76562499938548711, 101.5914258081833879 ) ) ;
#10015=ORIENTED_EDGE ( 'NONE', *, *, #27, .T. ) ;
#10019=CARTESIAN_POINT ( 'NONE',  ( -79.39999999999999147, -33.37500000000000000, 99.99999999999998579 ) ) ;
#10027=DIRECTION ( 'NONE',  ( -0.000000000000000000, -1.000000000000000000, -0.000000000000000000 ) ) ;
#10028=CARTESIAN_POINT ( 'NONE',  ( -80.90000000000000568, -34.64999999999999858, 97.40192378864668399 ) ) ;
#10053=CARTESIAN_POINT ( 'NONE',  ( -85.40000000000000568, -35.36739040097838682, 98.90809659374338025 ) ) ;
#10054=CARTESIAN_POINT ( 'NONE',  ( -82.39999999999999147, -30.81562499938548427, 96.81714838363319586 ) ) ;
#10067=CARTESIAN_POINT ( 'NONE',  ( -81.02178482187500208, -30.74062499938548498, 97.61286128772489690 ) ) ;
#10075=EDGE_CURVE ( 'NONE', #9639, #6974, #7684, .T. ) ;
#10079=CARTESIAN_POINT ( 'NONE',  ( -85.40000000000000568, -31.76249999999999929, 101.7320508075688679 ) ) ;
#10087=ORIENTED_EDGE ( 'NONE', *, *, #9148, .F. ) ;
#10089=FACE_OUTER_BOUND ( 'NONE', #4667, .T. ) ;
#10090=CARTESIAN_POINT ( 'NONE',  ( -79.39999999999999147, -33.35624999877096997, 101.7320508075688537 ) ) ;
#10092=CARTESIAN_POINT ( 'NONE',  ( -79.64356964374999848, -34.52812499938548285, 99.99999999999998579 ) ) ;
#10098=CARTESIAN_POINT ( 'NONE',  ( -82.39999999999999147, -33.17812499938548854, 103.1828516163667899 ) ) ;
#10102=CARTESIAN_POINT ( 'NONE',  ( -83.20384757729335945, -32.60759618943233562, 102.9999999999999858 ) ) ;
#10105=CARTESIAN_POINT ( 'NONE',  ( -79.39999999999999147, -30.63750000000000284, 98.26794919243110371 ) ) ;
#10116=CARTESIAN_POINT ( 'NONE',  ( -82.39999999999999147, -33.71249999999999858, 96.53589838486223584 ) ) ;
#10123=CARTESIAN_POINT ( 'NONE',  ( -80.90000000000000568, -30.29606250001229384, 102.5980762113533018 ) ) ;
#10127=CARTESIAN_POINT ( 'NONE',  ( -83.90000000000000568, -34.51874999877097139, 97.40192378864668399 ) ) ;
#10128=CARTESIAN_POINT ( 'NONE',  ( -82.40000000000001990, -32.75624999877096855, 97.00000000000000000 ) ) ;
#10134=ORIENTED_EDGE ( 'NONE', *, *, #5825, .T. ) ;
#10140=ORIENTED_EDGE ( 'NONE', *, *, #9647, .T. ) ;
#10148=CARTESIAN_POINT ( 'NONE',  ( -85.40000000000000568, -34.89374999877097139, 99.99999999999998579 ) ) ;
#10149=CARTESIAN_POINT ( 'NONE',  ( -85.15643035624999868, -30.29062499938548925, 98.40857419181659793 ) ) ;
#10160=CARTESIAN_POINT ( 'NONE',  ( -79.64356964374998427, -32.12812499938548427, 98.40857419181659793 ) ) ;
#10171=CARTESIAN_POINT ( 'NONE',  ( -79.39999999999999147, -32.43750000000000000, 98.26794919243110371 ) ) ;
#10174=CARTESIAN_POINT ( 'NONE',  ( -84.69814140657796031, -35.23021079535107702, 98.07164679703846843 ) ) ;
#10183=CARTESIAN_POINT ( 'NONE',  ( -85.15643035625001289, -31.94062499938548427, 99.99999999999998579 ) ) ;
#10190=CARTESIAN_POINT ( 'NONE',  ( -83.90000000000000568, -31.72500000000000142, 102.5980762113533018 ) ) ;
#10191=CARTESIAN_POINT ( 'NONE',  ( -79.64356964375001269, -34.82812499938548711, 98.40857419181659793 ) ) ;
#10200=ADVANCED_FACE ( 'NONE', ( #2495 ), #853, .T. ) ;
#10203=EDGE_CURVE ( 'NONE', #15015, #14886, #15935, .T. ) ;
#10207=EDGE_CURVE ( 'NONE', #10587, #11515, #18732, .T. ) ;
#10214=CARTESIAN_POINT ( 'NONE',  ( -83.20384757729334524, -30.54240381056766651, 96.99999999999997158 ) ) ;
#10217=CARTESIAN_POINT ( 'NONE',  ( -85.40000000000000568, -33.59606250001230165, 99.99999999999998579 ) ) ;
#10221=CARTESIAN_POINT ( 'NONE',  ( -79.64356964375001269, -32.12812499938548427, 98.40857419181659793 ) ) ;
#10222=CYLINDRICAL_SURFACE ( 'NONE', #17042, 3.000000000000002665 ) ;
#10237=CARTESIAN_POINT ( 'NONE',  ( -82.39999999999999147, -34.97812499938547859, 103.1828516163667899 ) ) ;
#10250=CARTESIAN_POINT ( 'NONE',  ( -85.40000000000000568, -34.03124999877096712, 98.26794919243111792 ) ) ;
#10251=CARTESIAN_POINT ( 'NONE',  ( -79.64356964375001269, -33.21562499938548996, 101.5914258081833879 ) ) ;
#10262=CARTESIAN_POINT ( 'NONE',  ( -83.77821517812500929, -33.81562499938548427, 97.61286128772489690 ) ) ;
#10273=CARTESIAN_POINT ( 'NONE',  ( -82.40000000000000568, -34.38749999999999574, 102.9999999999999858 ) ) ;
#10275=CARTESIAN_POINT ( 'NONE',  ( -85.40000000000000568, -32.28750000000000142, 98.26794919243111792 ) ) ;
#10284=CARTESIAN_POINT ( 'NONE',  ( -82.40000000000000568, -34.78124999877096712, 102.9999999999999858 ) ) ;
#10286=CARTESIAN_POINT ( 'NONE',  ( -82.39999999999999147, -30.70312499938548711, 96.81714838363319586 ) ) ;
#10292=CARTESIAN_POINT ( 'NONE',  ( -82.39999999999999147, -30.78750000000000497, 103.4641016151377499 ) ) ;
#10293=CARTESIAN_POINT ( 'NONE',  ( -82.39999999999999147, -32.36250000000000426, 96.99999999999998579 ) ) ;
#10307=CARTESIAN_POINT ( 'NONE',  ( -82.40000000000000568, -34.78124999877096712, 102.9999999999999858 ) ) ;
#10316=CARTESIAN_POINT ( 'NONE',  ( -85.40000000000000568, -31.30856250001229668, 101.7320508075688679 ) ) ;
#10318=CARTESIAN_POINT ( 'NONE',  ( -85.15643035625001289, -31.04062499938548569, 99.99999999999998579 ) ) ;
#10319=CARTESIAN_POINT ( 'NONE',  ( -81.59615242270662350, -32.83259618943233704, 96.99999999999998579 ) ) ;
#10334=VERTEX_POINT ( 'NONE', #16272 ) ;
#10335=CARTESIAN_POINT ( 'NONE',  ( -83.20384757729338787, -32.10134618820330132, 102.9999999999999858 ) ) ;
#10339=CARTESIAN_POINT ( 'NONE',  ( -79.39999999999999147, -32.42268749875867684, 99.99999999999998579 ) ) ;
#10340=CARTESIAN_POINT ( 'NONE',  ( -81.02178482187500208, -34.60312499938549280, 102.3871387122750889 ) ) ;
#10351=CARTESIAN_POINT ( 'NONE',  ( -83.77821517812500929, -33.66562499938548569, 102.3871387122750889 ) ) ;
#10363=CARTESIAN_POINT ( 'NONE',  ( -83.90000000000000568, -32.77499999999999858, 97.40192378864668399 ) ) ;
#10364=CARTESIAN_POINT ( 'NONE',  ( -83.90000000000000568, -32.11874999877097281, 102.5980762113533018 ) ) ;
#10369=ORIENTED_EDGE ( 'NONE', *, *, #8001, .T. ) ;
#10374=( BOUNDED_CURVE ( )  B_SPLINE_CURVE ( 2, ( #18785, #17219, #3542, #8234, #6577, #2463, #13990, #5314, #12622 ),
 .UNSPECIFIED., .F., .F. ) 
 B_SPLINE_CURVE_WITH_KNOTS ( ( 3, 2, 2, 2, 3 ),
 ( 0.6041666666666666297, 0.6111111111111111605, 0.6250000000000000000, 0.6388888888888888395, 0.6458333333333332593 ),
 .UNSPECIFIED. ) 
 CURVE ( )  GEOMETRIC_REPRESENTATION_ITEM ( )  RATIONAL_B_SPLINE_CURVE ( ( 0.9330127018922192983, 0.9330127018922187432, 1.000000000000000000, 0.8660254037844387076, 1.000000000000000000, 0.8660254037844387076, 1.000000000000000000, 0.9330127018922198534, 0.9330127018922192983 ) ) 
 REPRESENTATION_ITEM ( '' )  );
#10377=CARTESIAN_POINT ( 'NONE',  ( -79.64356964375001269, -31.30312499938548854, 101.5914258081833879 ) ) ;
#10383=CARTESIAN_POINT ( 'NONE',  ( -79.39999999999999147, -31.16250000000000497, 101.7320508075688537 ) ) ;
#10405=CARTESIAN_POINT ( 'NONE',  ( -83.90000000000000568, -31.42106250001229384, 97.40192378864668399 ) ) ;
#10408=CARTESIAN_POINT ( 'NONE',  ( -79.64356964375001269, -31.30312499938548854, 101.5914258081833879 ) ) ;
#10412=CARTESIAN_POINT ( 'NONE',  ( -82.40000000000000568, -30.00000000000000355, 99.99999999999998579 ) ) ;
#10413=CYLINDRICAL_SURFACE ( 'NONE', #6953, 3.000000000000002665 ) ;
#10430=CARTESIAN_POINT ( 'NONE',  ( -80.90000000000000568, -30.69768749875868252, 102.5980762113533018 ) ) ;
#10431=CARTESIAN_POINT ( 'NONE',  ( -82.39999999999999147, -32.84062499938548996, 103.1828516163667899 ) ) ;
#10445=CARTESIAN_POINT ( 'NONE',  ( -82.39999999999999147, -33.17812499938548854, 103.1828516163667899 ) ) ;
#10446=ORIENTED_EDGE ( 'NONE', *, *, #14324, .T. ) ;
#10456=CARTESIAN_POINT ( 'NONE',  ( -85.40000000000000568, -34.01250000000000284, 101.7320508075688679 ) ) ;
#10458=CARTESIAN_POINT ( 'NONE',  ( -80.90000000000000568, -32.04374999877096997, 102.5980762113533018 ) ) ;
#10463=ORIENTED_EDGE ( 'NONE', *, *, #18600, .T. ) ;
#10467=CARTESIAN_POINT ( 'NONE',  ( -82.39999999999999147, -31.40624999877096712, 96.99999999999998579 ) ) ;
#10469=CARTESIAN_POINT ( 'NONE',  ( -79.64356964375001269, -30.77812499938548285, 98.40857419181659793 ) ) ;
#10477=CARTESIAN_POINT ( 'NONE',  ( -79.39999999999999147, -31.12500000000000355, 99.99999999999998579 ) ) ;
#10494=CARTESIAN_POINT ( 'NONE',  ( -82.40000000000000568, -30.00000000000000355, 96.99999999999998579 ) ) ;
#10501=CARTESIAN_POINT ( 'NONE',  ( -85.40000000000000568, -31.75856250001229242, 101.7320508075688679 ) ) ;
#10505=CARTESIAN_POINT ( 'NONE',  ( -82.39999999999999147, -32.50312499938548427, 96.81714838363319586 ) ) ;
#10517=CARTESIAN_POINT ( 'NONE',  ( -82.40000000000001990, -33.26250000000000284, 97.00000000000000000 ) ) ;
#10528=CARTESIAN_POINT ( 'NONE',  ( -80.90000000000000568, -31.14768749875868181, 102.5980762113533018 ) ) ;
#10530=CARTESIAN_POINT ( 'NONE',  ( -85.15643035625001289, -34.75312499938548427, 99.99999999999998579 ) ) ;
#10540=AXIS2_PLACEMENT_3D ( 'NONE', #7341, #19270, #11738 ) ;
#10547=CARTESIAN_POINT ( 'NONE',  ( -79.64356964374998427, -33.02812499938548285, 98.40857419181659793 ) ) ;
#10549=ORIENTED_EDGE ( 'NONE', *, *, #5654, .F. ) ;
#10554=CARTESIAN_POINT ( 'NONE',  ( -82.40000000000000568, -31.63124999877096855, 102.9999999999999858 ) ) ;
#10559=CARTESIAN_POINT ( 'NONE',  ( -84.69814161231455785, -35.00052329606839407, 98.07164704222793716 ) ) ;
#10560=CARTESIAN_POINT ( 'NONE',  ( -85.40000000000000568, -32.23124999877096997, 98.26794919243111792 ) ) ;
#10563=CARTESIAN_POINT ( 'NONE',  ( -82.40000000000000568, -30.00000000000000355, 99.99999999999998579 ) ) ;
#10572=CARTESIAN_POINT ( 'NONE',  ( -79.64356964374999848, -30.36562499938548498, 99.99999999999998579 ) ) ;
#10577=CARTESIAN_POINT ( 'NONE',  ( -85.40000000000000568, -31.80000000000000071, 99.99999999999998579 ) ) ;
#10578=CARTESIAN_POINT ( 'NONE',  ( -85.40000000000000568, -30.03750000000000497, 98.26794919243111792 ) ) ;
#10587=VERTEX_POINT ( 'NONE', #3073 ) ;
#10597=CARTESIAN_POINT ( 'NONE',  ( -83.81335597582008745, -34.99989732956152721, 102.6513159617165201 ) ) ;
#10600=CARTESIAN_POINT ( 'NONE',  ( -85.40000000000000568, -33.18356250001228602, 98.26794919243111792 ) ) ;
#10601=( BOUNDED_CURVE ( )  B_SPLINE_CURVE ( 2, ( #7965, #750, #1813, #6705, #12650, #15294, #9233, #15196, #16763 ),
 .UNSPECIFIED., .F., .F. ) 
 B_SPLINE_CURVE_WITH_KNOTS ( ( 3, 2, 2, 2, 3 ),
 ( 0.4791666666666666297, 0.4861111111111111049, 0.5000000000000000000, 0.5138888888888888395, 0.5208333333333333703 ),
 .UNSPECIFIED. ) 
 CURVE ( )  GEOMETRIC_REPRESENTATION_ITEM ( )  RATIONAL_B_SPLINE_CURVE ( ( 0.9330127018922194093, 0.9330127018922190762, 1.000000000000000000, 0.8660254037844387076, 1.000000000000000000, 0.8660254037844387076, 1.000000000000000000, 0.9330127018922187432, 0.9330127018922192983 ) ) 
 REPRESENTATION_ITEM ( '' )  );
#10623=CARTESIAN_POINT ( 'NONE',  ( -82.39999999999999147, -30.73518749875867684, 103.4641016151377499 ) ) ;
#10625=CARTESIAN_POINT ( 'NONE',  ( -85.15643035624999868, -32.46562499938548996, 101.5914258081833879 ) ) ;
#10637=CARTESIAN_POINT ( 'NONE',  ( -81.02178482187500208, -32.54062499938548569, 97.61286128772489690 ) ) ;
#10643=CARTESIAN_POINT ( 'NONE',  ( -82.39999999999999147, -32.30624999877096570, 96.99999999999998579 ) ) ;
#10646=CARTESIAN_POINT ( 'NONE',  ( -82.39999999999999147, -33.48750000000000426, 103.4641016151377499 ) ) ;
#10648=CARTESIAN_POINT ( 'NONE',  ( -82.39999999999999147, -31.18124999877096926, 103.4641016151377499 ) ) ;
#10649=CARTESIAN_POINT ( 'NONE',  ( -82.39999999999999147, -32.58750000000000568, 102.9999999999999858 ) ) ;
#10650=CARTESIAN_POINT ( 'NONE',  ( -83.77821517812500929, -35.12812499938548427, 102.3871387122750889 ) ) ;
#10652=DIRECTION ( 'NONE',  ( 0.000000000000000000, 1.000000000000000000, 0.000000000000000000 ) ) ;
#10662=VERTEX_POINT ( 'NONE', #4544 ) ;
#10665=CARTESIAN_POINT ( 'NONE',  ( -85.40000000000000568, -31.76249999999999929, 101.7320508075688679 ) ) ;
#10678=EDGE_CURVE ( 'NONE', #6974, #7760, #17931, .T. ) ;
#10683=CARTESIAN_POINT ( 'NONE',  ( -79.64356964374999848, -31.82812499938548356, 99.99999999999998579 ) ) ;
#10688=CARTESIAN_POINT ( 'NONE',  ( -79.42451116572152614, -34.99876810435319641, 100.5066497421356786 ) ) ;
#10691=CARTESIAN_POINT ( 'NONE',  ( -82.39999999999999147, -32.36250000000000426, 96.99999999999997158 ) ) ;
#10692=CARTESIAN_POINT ( 'NONE',  ( -80.90000000000000568, -34.19606250001229597, 97.40192378864668399 ) ) ;
#10695=CARTESIAN_POINT ( 'NONE',  ( -81.02178482187500208, -32.35312499938548569, 102.3871387122750889 ) ) ;
#10706=CARTESIAN_POINT ( 'NONE',  ( -82.40000000000000568, -30.00000000000000355, 99.99999999999998579 ) ) ;
#10718=CARTESIAN_POINT ( 'NONE',  ( -79.39999999999999147, -31.93518749875867968, 98.26794919243110371 ) ) ;
#10736=CARTESIAN_POINT ( 'NONE',  ( -85.40000000000000568, -30.88124999877096855, 98.26794919243111792 ) ) ;
#10738=ORIENTED_EDGE ( 'NONE', *, *, #7559, .T. ) ;
#10742=CARTESIAN_POINT ( 'NONE',  ( -83.90000000000000568, -30.76874999877097139, 102.5980762113533018 ) ) ;
#10744=CARTESIAN_POINT ( 'NONE',  ( -80.90000000000000568, -32.79374999877096997, 97.40192378864668399 ) ) ;
#10745=DIRECTION ( 'NONE',  ( 0.000000000000000000, 1.000000000000000000, 0.000000000000000000 ) ) ;
#10748=DIRECTION ( 'NONE',  ( 0.000000000000000000, 0.000000000000000000, 1.000000000000000000 ) ) ;
#10749=DIRECTION ( 'NONE',  ( 0.000000000000000000, 0.000000000000000000, -1.000000000000000000 ) ) ;
#10755=DIRECTION ( 'NONE',  ( 0.000000000000000000, 0.000000000000000000, 1.000000000000000000 ) ) ;
#10769=FACE_OUTER_BOUND ( 'NONE', #12683, .T. ) ;
#10779=CARTESIAN_POINT ( 'NONE',  ( -81.02178482187500208, -30.85312499938548569, 97.61286128772489690 ) ) ;
#10789=CARTESIAN_POINT ( 'NONE',  ( -81.02178482187500208, -31.00312499938548783, 102.3871387122750889 ) ) ;
#10811=CARTESIAN_POINT ( 'NONE',  ( -84.69814161231455785, -35.39821079482706523, 98.07164704222793716 ) ) ;
#10828=EDGE_CURVE ( 'NONE', #6176, #2034, #12670, .T. ) ;
#10837=CARTESIAN_POINT ( 'NONE',  ( -82.39999999999999147, -34.83749999999999858, 103.4641016151377499 ) ) ;
#10838=CARTESIAN_POINT ( 'NONE',  ( -85.40000000000000568, -34.93124999877096570, 98.26794919243111792 ) ) ;
#10852=CARTESIAN_POINT ( 'NONE',  ( -82.39999999999999147, -31.91249999999999787, 96.99999999999998579 ) ) ;
#10854=ORIENTED_EDGE ( 'NONE', *, *, #5113, .T. ) ;
#10859=EDGE_LOOP ( 'NONE', ( #16913, #8670, #17405, #2232 ) ) ;
#10867=AXIS2_PLACEMENT_3D ( 'NONE', #6481, #7644, #9399 ) ;
#10874=CARTESIAN_POINT ( 'NONE',  ( -82.39999999999999147, -31.01249999999999929, 96.99999999999998579 ) ) ;
#10876=CARTESIAN_POINT ( 'NONE',  ( -85.15643035625001289, -32.50312499938548427, 99.99999999999998579 ) ) ;
#10887=CARTESIAN_POINT ( 'NONE',  ( -83.77821517812500929, -30.32812499938548711, 97.61286128772489690 ) ) ;
#10898=EDGE_CURVE ( 'NONE', #2034, #14891, #14407, .T. ) ;
#10905=CARTESIAN_POINT ( 'NONE',  ( -79.39999999999999147, -32.45624999877097139, 101.7320508075688537 ) ) ;
#10910=CARTESIAN_POINT ( 'NONE',  ( -83.90000000000000568, -33.47268749875867400, 102.5980762113533018 ) ) ;
#10913=CARTESIAN_POINT ( 'NONE',  ( -83.20384757729337366, -34.35134618820330843, 103.0000000000000000 ) ) ;
#10914=FACE_OUTER_BOUND ( 'NONE', #3408, .T. ) ;
#10919=VERTEX_POINT ( 'NONE', #8644 ) ;
#10924=ADVANCED_FACE ( 'NONE', ( #7093 ), #12046, .T. ) ;
#10925=CARTESIAN_POINT ( 'NONE',  ( -82.39999999999999147, -34.30312499938548143, 96.81714838363319586 ) ) ;
#10934=CARTESIAN_POINT ( 'NONE',  ( -83.90000000000000568, -31.21874999877097068, 102.5980762113533018 ) ) ;
#10937=CARTESIAN_POINT ( 'NONE',  ( -79.39999999999999147, -31.51874999877096784, 99.99999999999998579 ) ) ;
#10938=CARTESIAN_POINT ( 'NONE',  ( -83.90000000000000568, -34.51874999877097139, 97.40192378864668399 ) ) ;
#10940=ADVANCED_FACE ( 'NONE', ( #2403 ), #957, .T. ) ;
#10942=ORIENTED_EDGE ( 'NONE', *, *, #10956, .F. ) ;
#10956=EDGE_CURVE ( 'NONE', #16985, #8815, #9943, .T. ) ;
#10965=ORIENTED_EDGE ( 'NONE', *, *, #11966, .F. ) ;
#10968=CARTESIAN_POINT ( 'NONE',  ( -82.40000000000000568, -34.10624999877096997, 96.99999999999998579 ) ) ;
#10969=CARTESIAN_POINT ( 'NONE',  ( -79.64356964374999848, -30.92812499938548498, 99.99999999999998579 ) ) ;
#10973=CARTESIAN_POINT ( 'NONE',  ( -81.29668248076569625, -34.99857710348262430, 102.8092562322720198 ) ) ;
#10979=CARTESIAN_POINT ( 'NONE',  ( -85.15643035625001289, -31.64062499938548356, 98.40857419181659793 ) ) ;
#10987=ORIENTED_EDGE ( 'NONE', *, *, #10898, .F. ) ;
#10995=CARTESIAN_POINT ( 'NONE',  ( -82.40000000000000568, -35.00000000000000000, 99.99999999999998579 ) ) ;
#11001=CARTESIAN_POINT ( 'NONE',  ( -85.40000000000000568, -34.44768749875867542, 99.99999999999998579 ) ) ;
#11010=EDGE_CURVE ( 'NONE', #6176, #12057, #14409, .T. ) ;
#11017=CARTESIAN_POINT ( 'NONE',  ( -81.02178482187500208, -34.04062499938548569, 102.3871387122750889 ) ) ;
#11023=CARTESIAN_POINT ( 'NONE',  ( -83.90000000000000568, -30.76874999877097139, 102.5980762113533018 ) ) ;
#11029=CARTESIAN_POINT ( 'NONE',  ( -85.40000000000000568, -31.74374999877096926, 99.99999999999998579 ) ) ;
#11031=CARTESIAN_POINT ( 'NONE',  ( -80.90000000000000568, -35.19374999877096855, 102.5980762113533018 ) ) ;
#11032=CARTESIAN_POINT ( 'NONE',  ( -85.40000000000000568, -32.25000000000000000, 99.99999999999998579 ) ) ;
#11053=CARTESIAN_POINT ( 'NONE',  ( -83.90000000000000568, -34.57106250001229597, 97.40192378864668399 ) ) ;
#11067=CARTESIAN_POINT ( 'NONE',  ( -85.15643035624999868, -31.11562499938548854, 101.5914258081833879 ) ) ;
#11071=CARTESIAN_POINT ( 'NONE',  ( -81.28560337669112812, -35.00129552118395537, 97.20965008810277652 ) ) ;
#11075=AXIS2_PLACEMENT_3D ( 'NONE', #18464, #4693, #15042 ) ;
#11077=CARTESIAN_POINT ( 'NONE',  ( -79.64356964374998427, -31.79062499938548925, 98.40857419181659793 ) ) ;
#11091=ORIENTED_EDGE ( 'NONE', *, *, #16886, .T. ) ;
#11095=CARTESIAN_POINT ( 'NONE',  ( -82.40000000000001990, -32.75624999877096855, 97.00000000000000000 ) ) ;
#11097=CARTESIAN_POINT ( 'NONE',  ( -79.39999999999999147, -34.63518749875868252, 98.26794919243110371 ) ) ;
#11099=CARTESIAN_POINT ( 'NONE',  ( -82.40000000000000568, -30.00000000000000355, 103.0000000000000000 ) ) ;
#11113=CARTESIAN_POINT ( 'NONE',  ( -82.39999999999999147, -33.62812499938549138, 103.1828516163667899 ) ) ;
#11114=CARTESIAN_POINT ( 'NONE',  ( -85.15643035624999868, -35.11426555956768425, 98.99674139749697588 ) ) ;
#11116=ORIENTED_EDGE ( 'NONE', *, *, #1511, .F. ) ;
#11118=CARTESIAN_POINT ( 'NONE',  ( -83.20384757729337366, -30.75134618820329990, 103.0000000000000000 ) ) ;
#11124=CARTESIAN_POINT ( 'NONE',  ( -85.40000000000000568, -32.19374999877096855, 99.99999999999998579 ) ) ;
#11125=CARTESIAN_POINT ( 'NONE',  ( -85.40000000000000568, -33.13124999877096855, 98.26794919243111792 ) ) ;
#11137=DIRECTION ( 'NONE',  ( -0.000000000000000000, 1.000000000000000000, -0.000000000000000000 ) ) ;
#11144=CARTESIAN_POINT ( 'NONE',  ( -79.39999999999999147, -33.80624999877097281, 101.7320508075688537 ) ) ;
#11153=CARTESIAN_POINT ( 'NONE',  ( -79.39999999999999147, -30.22500000000000142, 99.99999999999998579 ) ) ;
#11154=DIRECTION ( 'NONE',  ( -0.000000000000000000, -1.000000000000000000, -0.000000000000000000 ) ) ;
#11162=( BOUNDED_CURVE ( )  B_SPLINE_CURVE ( 2, ( #2368, #11458, #16144, #2757, #14666, #10090, #1202, #18989, #9899 ),
 .UNSPECIFIED., .F., .F. ) 
 B_SPLINE_CURVE_WITH_KNOTS ( ( 3, 2, 2, 2, 3 ),
 ( 0.5208333333333333703, 0.5277777777777777901, 0.5416666666666666297, 0.5555555555555555802, 0.5625000000000000000 ),
 .UNSPECIFIED. ) 
 CURVE ( )  GEOMETRIC_REPRESENTATION_ITEM ( )  RATIONAL_B_SPLINE_CURVE ( ( 0.9330127018922192983, 0.9330127018922198534, 1.000000000000000000, 0.8660254037844387076, 1.000000000000000000, 0.8660254037844387076, 1.000000000000000000, 0.9330127018922194093, 0.9330127018922194093 ) ) 
 REPRESENTATION_ITEM ( '' )  );
#11169=CARTESIAN_POINT ( 'NONE',  ( -83.77821517812500929, -33.77812499938548285, 102.3871387122750889 ) ) ;
#11178=VECTOR ( 'NONE', #12794, 1000.000000000000000 ) ;
#11180=CARTESIAN_POINT ( 'NONE',  ( -81.02178482187500208, -34.00312499938548427, 97.61286128772489690 ) ) ;
#11191=CARTESIAN_POINT ( 'NONE',  ( -82.39999999999999147, -33.03750000000000142, 103.4641016151377499 ) ) ;
#11199=CARTESIAN_POINT ( 'NONE',  ( -80.90000000000000568, -30.59606250001229100, 97.40192378864668399 ) ) ;
#11201=CARTESIAN_POINT ( 'NONE',  ( -85.40000000000000568, -35.34768749875867400, 99.99999999999998579 ) ) ;
#11217=CARTESIAN_POINT ( 'NONE',  ( -82.39999999999999147, -33.17812499938548854, 103.1828516163667899 ) ) ;
#11227=CARTESIAN_POINT ( 'NONE',  ( -80.90000000000000568, -31.44374999877096855, 97.40192378864668399 ) ) ;
#11228=CARTESIAN_POINT ( 'NONE',  ( -79.39999999999999147, -32.83124999877097139, 98.26794919243110371 ) ) ;
#11230=( BOUNDED_CURVE ( )  B_SPLINE_CURVE ( 2, ( #7624, #14681, #19191, #10105, #1858, #319, #6360, #4241, #13218 ),
 .UNSPECIFIED., .F., .F. ) 
 B_SPLINE_CURVE_WITH_KNOTS ( ( 3, 2, 2, 2, 3 ),
 ( 0.1041666666666666713, 0.1111111111111111049, 0.1250000000000000000, 0.1388888888888888951, 0.1458333333333333426 ),
 .UNSPECIFIED. ) 
 CURVE ( )  GEOMETRIC_REPRESENTATION_ITEM ( )  RATIONAL_B_SPLINE_CURVE ( ( 0.9330127018922194093, 0.9330127018922194093, 1.000000000000000000, 0.8660254037844387076, 1.000000000000000000, 0.8660254037844387076, 1.000000000000000000, 0.9330127018922194093, 0.9330127018922194093 ) ) 
 REPRESENTATION_ITEM ( '' )  );
#11241=CARTESIAN_POINT ( 'NONE',  ( -85.15643035625001289, -30.17812499938548498, 98.40857419181659793 ) ) ;
#11242=DIRECTION ( 'NONE',  ( 0.000000000000000000, 0.000000000000000000, -1.000000000000000000 ) ) ;
#11251=CARTESIAN_POINT ( 'NONE',  ( -79.39999999999999147, -33.78356250001230165, 98.26794919243110371 ) ) ;
#11255=CARTESIAN_POINT ( 'NONE',  ( -82.40000000000000568, -30.00000000000000355, 99.99999999999998579 ) ) ;
#11258=EDGE_LOOP ( 'NONE', ( #1496, #7833, #9237, #222, #10446, #18050, #9101, #10854, #3545, #17921, #14687, #1595, #4152, #5468, #4461, #12278, #3024, #17259, #9138, #18008, #7509, #9843, #15353, #12444, #8978, #7299 ) ) ;
#11262=CARTESIAN_POINT ( 'NONE',  ( -85.15643035624999868, -33.89062499938548711, 98.40857419181659793 ) ) ;
#11267=CARTESIAN_POINT ( 'NONE',  ( -83.77821517812500929, -35.01562499938548711, 102.3871387122750889 ) ) ;
#11269=CARTESIAN_POINT ( 'NONE',  ( -82.39999999999999147, -31.46249999999999858, 96.99999999999998579 ) ) ;
#11273=CARTESIAN_POINT ( 'NONE',  ( -85.15643035625001289, -33.85312499938549280, 99.99999999999998579 ) ) ;
#11285=CARTESIAN_POINT ( 'NONE',  ( -85.40000000000000568, -34.08749999999999858, 98.26794919243111792 ) ) ;
#11291=AXIS2_PLACEMENT_3D ( 'NONE', #4085, #5372, #14524 ) ;
#11293=CYLINDRICAL_SURFACE ( 'NONE', #11919, 3.000000000000002665 ) ;
#11306=CIRCLE ( 'NONE', #4445, 3.000000000000002665 ) ;
#11320=ORIENTED_EDGE ( 'NONE', *, *, #13166, .F. ) ;
#11326=CARTESIAN_POINT ( 'NONE',  ( -79.39999999999999147, -34.18124999877097281, 98.26794919243110371 ) ) ;
#11327=CARTESIAN_POINT ( 'NONE',  ( -83.77821517812500929, -31.97812499938548925, 102.3871387122750889 ) ) ;
#11338=CARTESIAN_POINT ( 'NONE',  ( -85.15643035625001289, -31.52812499938548285, 98.40857419181659793 ) ) ;
#11349=CARTESIAN_POINT ( 'NONE',  ( -85.40000000000000568, -29.95670094768209779, 101.9998975609119469 ) ) ;
#11361=CARTESIAN_POINT ( 'NONE',  ( -81.02178482187500208, -33.10312499938548569, 97.61286128772489690 ) ) ;
#11365=CARTESIAN_POINT ( 'NONE',  ( -82.39999999999999147, -32.95312499938548711, 96.81714838363319586 ) ) ;
#11370=CARTESIAN_POINT ( 'NONE',  ( -79.64356964374999848, -32.72812499938548569, 99.99999999999998579 ) ) ;
#11382=CARTESIAN_POINT ( 'NONE',  ( -85.40000000000000568, -33.56250000000000000, 101.7320508075688679 ) ) ;
#11385=CARTESIAN_POINT ( 'NONE',  ( -82.40000000000000568, -30.00000000000000355, 103.0000000000000000 ) ) ;
#11387=CIRCLE ( 'NONE', #11075, 7.500000000000020428 ) ;
#11393=CARTESIAN_POINT ( 'NONE',  ( -79.39999999999999147, -31.12106250001229313, 99.99999999999998579 ) ) ;
#11397=CARTESIAN_POINT ( 'NONE',  ( -83.20384757729338787, -34.53615380933862866, 97.00000000000000000 ) ) ;
#11398=CARTESIAN_POINT ( 'NONE',  ( -83.20384757729335945, -32.73615380933863150, 96.99999999999998579 ) ) ;
#11423=CARTESIAN_POINT ( 'NONE',  ( -79.39999999999999147, -33.80624999877097281, 101.7320508075688537 ) ) ;
#11424=CARTESIAN_POINT ( 'NONE',  ( -83.77821517812500929, -31.52812499938548996, 102.3871387122750889 ) ) ;
#11437=CARTESIAN_POINT ( 'NONE',  ( -81.02178482187500208, -32.24062499938548854, 102.3871387122750889 ) ) ;
#11439=EDGE_LOOP ( 'NONE', ( #18486, #16510, #897, #919 ) ) ;
#11448=CARTESIAN_POINT ( 'NONE',  ( -82.39999999999999147, -33.26250000000000284, 96.53589838486223584 ) ) ;
#11458=CARTESIAN_POINT ( 'NONE',  ( -81.59615242270662350, -33.22634618820330132, 96.99999999999998579 ) ) ;
#11460=CARTESIAN_POINT ( 'NONE',  ( -79.64356964375001269, -34.11562499938548854, 101.5914258081833879 ) ) ;
#11465=CARTESIAN_POINT ( 'NONE',  ( -79.64356964374999848, -34.41562499938548569, 99.99999999999998579 ) ) ;
#11471=CARTESIAN_POINT ( 'NONE',  ( -79.64356964374999848, -34.97812499938548569, 99.99999999999998579 ) ) ;
#11482=CARTESIAN_POINT ( 'NONE',  ( -85.40000000000000568, -34.46249999999999858, 101.7320508075688679 ) ) ;
#11491=CARTESIAN_POINT ( 'NONE',  ( -83.90000000000000568, -30.37106250001229313, 102.5980762113533018 ) ) ;
#11492=CARTESIAN_POINT ( 'NONE',  ( -82.40000000000000568, -34.61250000000001137, 97.00000000000000000 ) ) ;
#11496=CARTESIAN_POINT ( 'NONE',  ( -85.40000000000000568, -33.63750000000000284, 98.26794919243111792 ) ) ;
#11515=VERTEX_POINT ( 'NONE', #10007 ) ;
#11516=CARTESIAN_POINT ( 'NONE',  ( -83.90000000000000568, -32.26874999877097139, 97.40192378864668399 ) ) ;
#11521=CARTESIAN_POINT ( 'NONE',  ( -80.90000000000000568, -34.14374999877097139, 97.40192378864668399 ) ) ;
#11522=CARTESIAN_POINT ( 'NONE',  ( -82.39999999999999147, -30.59062499938548640, 103.1828516163667899 ) ) ;
#11533=CARTESIAN_POINT ( 'NONE',  ( -85.40000000000000568, -35.30624999877096570, 101.7320508075688821 ) ) ;
#11534=CARTESIAN_POINT ( 'NONE',  ( -81.02178482187500208, -31.79062499938548925, 102.3871387122750889 ) ) ;
#11535=ORIENTED_EDGE ( 'NONE', *, *, #14731, .F. ) ;
#11544=CARTESIAN_POINT ( 'NONE',  ( -80.90000000000000568, -31.05000000000000071, 97.40192378864668399 ) ) ;
#11554=CARTESIAN_POINT ( 'NONE',  ( -85.15643035625001289, -30.25312499938548783, 99.99999999999998579 ) ) ;
#11556=CARTESIAN_POINT ( 'NONE',  ( -83.77821517812500929, -33.32812499938548711, 102.3871387122750889 ) ) ;
#11561=CARTESIAN_POINT ( 'NONE',  ( -79.64356964374999848, -33.06562499938548427, 99.99999999999998579 ) ) ;
#11567=CARTESIAN_POINT ( 'NONE',  ( -79.64356964374998427, -34.11562499938548854, 101.5914258081833879 ) ) ;
#11577=CARTESIAN_POINT ( 'NONE',  ( -80.90000000000000568, -32.85000000000000142, 97.40192378864668399 ) ) ;
#11581=CARTESIAN_POINT ( 'NONE',  ( -85.40000000000000568, -30.45000000000000284, 99.99999999999998579 ) ) ;
#11584=CARTESIAN_POINT ( 'NONE',  ( -79.39999999999999147, -30.25856250001228887, 101.7320508075688537 ) ) ;
#11585=CARTESIAN_POINT ( 'NONE',  ( -79.39999999999999147, -34.68750000000000000, 98.26794919243110371 ) ) ;
#11587=CARTESIAN_POINT ( 'NONE',  ( -81.02178482187500208, -30.29062499938548569, 97.61286128772489690 ) ) ;
#11588=FACE_OUTER_BOUND ( 'NONE', #17985, .T. ) ;
#11600=VERTEX_POINT ( 'NONE', #17218 ) ;
#11608=CARTESIAN_POINT ( 'NONE',  ( -79.39999999999999147, -33.73124999877096997, 98.26794919243110371 ) ) ;
#11609=CARTESIAN_POINT ( 'NONE',  ( -81.02178482187500208, -32.20312499938548711, 97.61286128772489690 ) ) ;
#11610=CARTESIAN_POINT ( 'NONE',  ( -81.59615242270665192, -30.71115380933863648, 102.9999999999999858 ) ) ;
#11623=CARTESIAN_POINT ( 'NONE',  ( -83.77821517812500929, -32.01562499938548001, 97.61286128772489690 ) ) ;
#11632=CARTESIAN_POINT ( 'NONE',  ( -85.40000000000000568, -31.78124999877096712, 98.26794919243111792 ) ) ;
#11637=CARTESIAN_POINT ( 'NONE',  ( -82.39999999999999147, -32.81250000000000000, 96.53589838486223584 ) ) ;
#11641=CARTESIAN_POINT ( 'NONE',  ( -84.69814130370966154, -35.19739829545387977, 98.07164667444374118 ) ) ;
#11648=LINE ( 'NONE', #1013, #1180 ) ;
#11651=CARTESIAN_POINT ( 'NONE',  ( -79.64356964375001269, -31.75312499938548427, 101.5914258081833879 ) ) ;
#11654=ORIENTED_EDGE ( 'NONE', *, *, #10828, .F. ) ;
#11656=CARTESIAN_POINT ( 'NONE',  ( -79.64356964375001269, -34.45312499938548711, 101.5914258081833879 ) ) ;
#11662=ADVANCED_FACE ( 'NONE', ( #10914 ), #6530, .F. ) ;
#11671=CARTESIAN_POINT ( 'NONE',  ( -85.40000000000000568, -34.89374999877097139, 99.99999999999998579 ) ) ;
#11676=CARTESIAN_POINT ( 'NONE',  ( -83.90000000000000568, -30.37500000000000355, 102.5980762113533018 ) ) ;
#11679=CARTESIAN_POINT ( 'NONE',  ( -80.90000000000000568, -31.94606250001229242, 97.40192378864668399 ) ) ;
#11680=CARTESIAN_POINT ( 'NONE',  ( -81.59615242270665192, -34.81740381056767575, 103.0000000000000000 ) ) ;
#11682=CARTESIAN_POINT ( 'NONE',  ( -83.77821517812500929, -31.41562499938548569, 102.3871387122750889 ) ) ;
#11703=CARTESIAN_POINT ( 'NONE',  ( -79.39999999999999147, -30.62268749875867968, 99.99999999999998579 ) ) ;
#11705=CARTESIAN_POINT ( 'NONE',  ( -83.77821517812500929, -33.92812499938548854, 97.61286128772489690 ) ) ;
#11717=CARTESIAN_POINT ( 'NONE',  ( -81.02178482187500208, -34.04062499938548569, 102.3871387122750889 ) ) ;
#11729=CARTESIAN_POINT ( 'NONE',  ( -82.39999999999999147, -31.91250000000000497, 96.53589838486223584 ) ) ;
#11738=DIRECTION ( 'NONE',  ( 1.000000000000000000, 0.000000000000000000, 0.000000000000000000 ) ) ;
#11744=CARTESIAN_POINT ( 'NONE',  ( -85.15643035625001289, -30.59062499938548285, 99.99999999999998579 ) ) ;
#11750=CARTESIAN_POINT ( 'NONE',  ( -79.39999999999999147, -32.02500000000000568, 99.99999999999998579 ) ) ;
#11751=EDGE_CURVE ( 'NONE', #6735, #6176, #4578, .T. ) ;
#11765=LINE ( 'NONE', #10494, #886 ) ;
#11773=CARTESIAN_POINT ( 'NONE',  ( -82.39999999999999147, -32.35856250001229739, 96.53589838486223584 ) ) ;
#11779=CARTESIAN_POINT ( 'NONE',  ( -82.39999999999999147, -31.60312499938548569, 96.81714838363319586 ) ) ;
#11780=CARTESIAN_POINT ( 'NONE',  ( -83.20384757729337366, -32.55134618820330417, 103.0000000000000000 ) ) ;
#11799=ADVANCED_FACE ( 'NONE', ( #11588 ), #10222, .T. ) ;
#11806=CARTESIAN_POINT ( 'NONE',  ( -79.39999999999999147, -31.03518749875868110, 98.26794919243110371 ) ) ;
#11807=CARTESIAN_POINT ( 'NONE',  ( -79.64356964375001269, -32.69062499938548427, 98.40857419181659793 ) ) ;
#11811=CARTESIAN_POINT ( 'NONE',  ( -82.40000000000000568, -33.03750000000000142, 102.9999999999999858 ) ) ;
#11818=CARTESIAN_POINT ( 'NONE',  ( -81.02178482187500208, -34.34062499938548285, 97.61286128772489690 ) ) ;
#11829=CARTESIAN_POINT ( 'NONE',  ( -79.39999999999999147, -32.96250000000000568, 101.7320508075688537 ) ) ;
#11830=CARTESIAN_POINT ( 'NONE',  ( -85.40000000000000568, -30.88124999877097210, 98.26794919243111792 ) ) ;
#11831=DIRECTION ( 'NONE',  ( 0.000000000000000000, 0.000000000000000000, 1.000000000000000000 ) ) ;
#11840=CARTESIAN_POINT ( 'NONE',  ( -81.02178482187500208, -32.09062499938548285, 97.61286128772489690 ) ) ;
#11845=CARTESIAN_POINT ( 'NONE',  ( -82.40000000000000568, -31.68750000000000711, 102.9999999999999858 ) ) ;
#11846=CARTESIAN_POINT ( 'NONE',  ( -79.39999999999999147, -31.53750000000000497, 98.26794919243110371 ) ) ;
#11861=DIRECTION ( 'NONE',  ( -0.000000000000000000, 1.000000000000000000, -0.000000000000000000 ) ) ;
#11866=CARTESIAN_POINT ( 'NONE',  ( -81.59615242270662350, -30.97634618820330488, 96.99999999999998579 ) ) ;
#11868=CARTESIAN_POINT ( 'NONE',  ( -79.39999999999999147, -31.53356250001228744, 98.26794919243110371 ) ) ;
#11872=CARTESIAN_POINT ( 'NONE',  ( -85.15643035624999868, -31.52812499938547930, 98.40857419181659793 ) ) ;
#11875=EDGE_CURVE ( 'NONE', #4909, #1155, #9305, .T. ) ;
#11895=CARTESIAN_POINT ( 'NONE',  ( -79.39999999999999147, -32.46018749875867826, 101.7320508075688537 ) ) ;
#11896=CARTESIAN_POINT ( 'NONE',  ( -82.39999999999999147, -33.06562499938548427, 96.81714838363319586 ) ) ;
#11909=CARTESIAN_POINT ( 'NONE',  ( -79.64356964374998427, -34.45312499938548711, 101.5914258081833879 ) ) ;
#11919=AXIS2_PLACEMENT_3D ( 'NONE', #954, #13928, #3677 ) ;
#11922=CARTESIAN_POINT ( 'NONE',  ( -80.90000000000000568, -34.20000000000000284, 97.40192378864668399 ) ) ;
#11923=CARTESIAN_POINT ( 'NONE',  ( -85.40000000000000568, -31.29374999877096997, 99.99999999999998579 ) ) ;
#11933=( BOUNDED_CURVE ( )  B_SPLINE_CURVE ( 2, ( #7498, #16388, #3331, #7207, #16298, #2907, #7300, #13257, #8769 ),
 .UNSPECIFIED., .F., .F. ) 
 B_SPLINE_CURVE_WITH_KNOTS ( ( 3, 2, 2, 2, 3 ),
 ( 0.02083333333333332871, 0.02777777777777777624, 0.04166666666666666435, 0.05555555555555555247, 0.06250000000000002776 ),
 .UNSPECIFIED. ) 
 CURVE ( )  GEOMETRIC_REPRESENTATION_ITEM ( )  RATIONAL_B_SPLINE_CURVE ( ( 0.9330127018922191873, 0.9330127018922191873, 1.000000000000000000, 0.8660254037844387076, 1.000000000000000000, 0.8660254037844387076, 1.000000000000000000, 0.9330127018922190762, 0.9330127018922194093 ) ) 
 REPRESENTATION_ITEM ( '' )  );
#11936=CARTESIAN_POINT ( 'NONE',  ( -85.15643035624999868, -31.45312499938548356, 101.5914258081833879 ) ) ;
#11940=ORIENTED_EDGE ( 'NONE', *, *, #13417, .F. ) ;
#11942=CARTESIAN_POINT ( 'NONE',  ( -83.90000000000000568, -31.87500000000000000, 97.40192378864668399 ) ) ;
#11953=CARTESIAN_POINT ( 'NONE',  ( -82.39999999999999147, -31.40624999877096712, 96.99999999999998579 ) ) ;
#11957=CARTESIAN_POINT ( 'NONE',  ( -85.40000000000000568, -34.91250000000000142, 101.7320508075688679 ) ) ;
#11961=CARTESIAN_POINT ( 'NONE',  ( -82.40000000000000568, -31.18124999877096926, 102.9999999999999858 ) ) ;
#11962=CARTESIAN_POINT ( 'NONE',  ( -79.39999999999999147, -32.47500000000000142, 99.99999999999998579 ) ) ;
#11963=CARTESIAN_POINT ( 'NONE',  ( -79.39999999999999147, -33.33356250001228460, 98.26794919243110371 ) ) ;
#11966=EDGE_CURVE ( 'NONE', #12057, #14891, #1331, .T. ) ;
#11969=CARTESIAN_POINT ( 'NONE',  ( -79.64356964374999848, -31.26562499938548356, 99.99999999999998579 ) ) ;
#11976=VERTEX_POINT ( 'NONE', #16662 ) ;
#11981=CYLINDRICAL_SURFACE ( 'NONE', #14560, 3.000000000000002665 ) ;
#11993=CARTESIAN_POINT ( 'NONE',  ( -80.90000000000000568, -32.04768749875867684, 102.5980762113533018 ) ) ;
#11994=CARTESIAN_POINT ( 'NONE',  ( -85.15643035625001289, -34.30312499938548854, 99.99999999999998579 ) ) ;
#11995=CARTESIAN_POINT ( 'NONE',  ( -79.39999999999999147, -31.53749999999999787, 98.26794919243110371 ) ) ;
#12006=CARTESIAN_POINT ( 'NONE',  ( -81.02178482187500208, -32.69062499938548427, 102.3871387122750889 ) ) ;
#12016=CARTESIAN_POINT ( 'NONE',  ( -80.90000000000000568, -33.89999999999999858, 102.5980762113533018 ) ) ;
#12018=CARTESIAN_POINT ( 'NONE',  ( -83.90000000000000568, -30.76874999877097139, 102.5980762113533018 ) ) ;
#12032=CARTESIAN_POINT ( 'NONE',  ( -79.64356964374999848, -31.26562499938548356, 99.99999999999998579 ) ) ;
#12037=CARTESIAN_POINT ( 'NONE',  ( -83.20384757729335945, -31.89240381056766793, 96.99999999999997158 ) ) ;
#12038=CARTESIAN_POINT ( 'NONE',  ( -79.39999999999999147, -30.71250000000000568, 101.7320508075688537 ) ) ;
#12046=( BOUNDED_SURFACE ( )  B_SPLINE_SURFACE ( 1, 2, ( 
 ( #8365, #15795, #3965, #15700, #12764, #2687, #9831, #6999, #13050, #11584, #10123, #18733, #11491, #17165, #8454, #854, #14604, #5253, #11199, #3770, #9737, #2303, #14317, #8268, #9932, #15890, #6910, #956, #12859, #18830, #5452, #2496, #11393, #17355, #5544, #17455, #16369, #10316, #3074, #63, #10405, #14797, #5730, #11868, #16467, #4353, #4546, #13235, #2792, #10501, #16273, #1619, #17750, #3168, #11679, #17934, #19311, #4449, #9034, #19209, #16565, #14998, #7570, #8743, #13524, #11773, #1424, #160, #2977, #14696, #7281, #2885, #8841, #6113, #12063, #14896, #1526, #8933, #7476, #7377, #13334, #9128, #18038, #15090, #13433, #5923, #4651, #10600, #5824, #6017, #1707, #11963, #4258, #16182, #17836, #7660, #19110, #17645, #10217, #1334, #6869, #13616, #18590, #11251, #625, #16659, #3632, #17022, #910, #2071, #12617, #9493, #14273, #8230, #10692, #5112, #8028, #6772, #15850, #3261, #9888, #17215, #5206, #6573, #11053, #12816, #12720, #12521, #15461, #2261, #13987, #2459, #17314, #18492, #6215, #259, #9595 ),
 ( #11349, #3820, #9789, #15559, #15751, #2173, #8130, #2357, #11153, #14082, #720, #6676, #17122, #5309, #8319, #9693, #15655, #3728, #14178, #813, #12162, #18692, #18781, #5406, #3921, #18129, #4746, #5599, #14553, #19164, #11544, #2638, #5688, #17412, #4212, #5777, #8705, #8603, #9986, #5879, #16236, #14655, #17506, #14457, #18976, #1089, #7047, #16327, #7238, #10079, #4117, #2841, #16037, #11729, #15941, #8798, #19261, #14367, #2543, #1193, #17599, #13005, #13193, #10275, #13099, #18879, #8505, #10171, #7148, #19069, #8415, #4406, #17697, #4312, #1386, #16134, #10363, #11637, #1004, #6959, #2744, #11829, #14753, #17796, #1290, #7333, #13286, #12911, #5501, #11448, #4025, #16614, #7431, #22, #9080, #10646, #9272, #4697, #17989, #15142, #15241, #2936, #7621, #314, #8990, #5972, #12016, #6070, #1855, #10456, #1669, #17893, #3315, #3220, #11922, #13481, #16420, #1758, #4893, #4501, #18276, #6265, #13573, #14952, #121, #7813, #7716, #1577, #3030, #9178, #7525, #10837, #6357, #4600, #14849, #8889, #10559 ),
 ( #212, #12118, #16520, #13676, #12210, #18180, #3123, #18089, #15046, #4803, #1474, #12309, #10742, #13388, #6168, #16707, #13769, #409, #6649, #13960, #15533, #5282, #6551, #18376, #5378, #3510, #12496, #602, #15331, #500, #11227, #2150, #10937, #18562, #3417, #884, #5178, #788, #11029, #12594, #12790, #14154, #8107, #8296, #7907, #9765, #14246, #9470, #6845, #13858, #11124, #18759, #17192, #17092, #18663, #16808, #3705, #18467, #14060, #3796, #5087, #4994, #9369, #15432, #16993, #3605, #1949, #6453, #15726, #694, #16904, #9671, #12405, #2045, #15632, #6743, #9566, #2237, #8004, #12690, #8203, #2332, #2432, #4285, #2818, #3997, #8775, #8391, #1164, #1361, #5754, #11608, #7123, #11423, #17383, #19236, #7305, #8677, #14630, #10250, #19042, #13262, #11521, #11326, #9862, #12980, #14725, #7212, #17291, #13076, #17482, #13165, #3894, #9962, #5665, #15822, #17577, #14342, #980, #4091, #4188, #17672, #10148, #7026, #16110, #16212, #6935, #16012, #1265, #15916, #12886, #1069, #14435, #18857, #5477, #10053, #2521 ),
 ( #8478, #8577, #18950, #19137, #2717, #2616, #5574, #14532, #11703, #3193, #10430, #10623, #19321, #8865, #16589, #16394, #7689, #4477, #9247, #11806, #4674, #6046, #10528, #9152, #5948, #3288, #15115, #1731, #14822, #13645, #17866, #1554, #286, #16496, #1450, #13366, #3004, #8960, #6237, #12185, #1828, #18153, #4775, #10718, #13549, #7788, #11993, #13742, #4382, #7502, #15211, #16682, #5852, #15023, #17961, #17775, #10339, #11895, #189, #16303, #6139, #2913, #7403, #4571, #12089, #14928, #7596, #13458, #18063, #93, #3098, #9058, #1643, #6424, #3392, #9440, #3480, #6715, #7882, #18440, #15306, #762, #14033, #16777, #10910, #13833, #12567, #2305, #9343, #15703, #3681, #5059, #12380, #16876, #12661, #18535, #18346, #1919, #8080, #475, #8269, #3771, #4968, #12285, #6333, #15406, #5255, #2016, #8177, #15505, #11001, #9539, #7976, #2120, #9646, #11097, #13932, #669, #571, #15607, #18249, #9738, #4867, #6526, #18634, #12472, #6618, #3579, #5151, #16968, #380, #17066, #2213, #14124, #11201, #17167, #10811 ) ),
 .UNSPECIFIED., .F., .F., .F. ) 
 B_SPLINE_SURFACE_WITH_KNOTS ( ( 2, 1, 1, 2 ),
 ( 3, 2, 2, 2, 2, 2, 2, 2, 2, 2, 2, 2, 2, 2, 2, 2, 2, 2, 2, 2, 2, 2, 2, 2, 2, 2, 2, 2, 2, 2, 2, 2, 2, 2, 2, 2, 2, 2, 2, 2, 2, 2, 2, 2, 2, 2, 2, 2, 2, 2, 2, 2, 2, 2, 2, 2, 2, 2, 2, 2, 2, 2, 2, 2, 2, 2, 2, 2, 3 ),
 ( -0.01000000000000000021, 0.000000000000000000, 1.000000000000000000, 1.010000000000000009 ),
 ( -0.009258785004222062215, 0.000000000000000000, 0.01388888888888888812, 0.02777777777777777624, 0.04166666666666666435, 0.05555555555555555247, 0.06944444444444444753, 0.08333333333333332871, 0.09722222222222222376, 0.1111111111111111049, 0.1250000000000000000, 0.1388888888888888951, 0.1527777777777777901, 0.1666666666666666574, 0.1805555555555555525, 0.1944444444444444475, 0.2083333333333333426, 0.2222222222222222099, 0.2361111111111111049, 0.2500000000000000000, 0.2638888888888888951, 0.2777777777777777901, 0.2916666666666666852, 0.3055555555555555802, 0.3194444444444444198, 0.3333333333333333148, 0.3472222222222222099, 0.3611111111111111049, 0.3750000000000000000, 0.3888888888888888951, 0.4027777777777777901, 0.4166666666666666852, 0.4305555555555555802, 0.4444444444444444198, 0.4583333333333333148, 0.4722222222222222099, 0.4861111111111111049, 0.5000000000000000000, 0.5138888888888888395, 0.5277777777777777901, 0.5416666666666666297, 0.5555555555555555802, 0.5694444444444444198, 0.5833333333333333703, 0.5972222222222222099, 0.6111111111111111605, 0.6250000000000000000, 0.6388888888888888395, 0.6527777777777777901, 0.6666666666666666297, 0.6805555555555555802, 0.6944444444444444198, 0.7083333333333333703, 0.7222222222222222099, 0.7361111111111111605, 0.7500000000000000000, 0.7638888888888888395, 0.7777777777777777901, 0.7916666666666666297, 0.8055555555555555802, 0.8194444444444444198, 0.8333333333333333703, 0.8472222222222222099, 0.8611111111111111605, 0.8750000000000000000, 0.8888888888888888395, 0.9027777777777777901, 0.9166666666666666297, 0.9258785004222062076 ),
 .UNSPECIFIED. ) 
 GEOMETRIC_REPRESENTATION_ITEM ( )  RATIONAL_B_SPLINE_SURFACE ( (
 ( 1.000000000000000000, 1.000000000000000000, 1.000000000000000000, 0.8660254037844387076, 1.000000000000000000, 0.8660254037844387076, 1.000000000000000000, 0.8660254037844387076, 1.000000000000000000, 0.8660254037844387076, 1.000000000000000000, 0.8660254037844387076, 1.000000000000000000, 0.8660254037844387076, 1.000000000000000000, 0.8660254037844387076, 1.000000000000000000, 0.8660254037844387076, 1.000000000000000000, 0.8660254037844387076, 1.000000000000000000, 0.8660254037844387076, 1.000000000000000000, 0.8660254037844387076, 1.000000000000000000, 0.8660254037844387076, 1.000000000000000000, 0.8660254037844387076, 1.000000000000000000, 0.8660254037844387076, 1.000000000000000000, 0.8660254037844387076, 1.000000000000000000, 0.8660254037844387076, 1.000000000000000000, 0.8660254037844387076, 1.000000000000000000, 0.8660254037844387076, 1.000000000000000000, 0.8660254037844387076, 1.000000000000000000, 0.8660254037844387076, 1.000000000000000000, 0.8660254037844387076, 1.000000000000000000, 0.8660254037844387076, 1.000000000000000000, 0.8660254037844387076, 1.000000000000000000, 0.8660254037844387076, 1.000000000000000000, 0.8660254037844387076, 1.000000000000000000, 0.8660254037844387076, 1.000000000000000000, 0.8660254037844387076, 1.000000000000000000, 0.8660254037844387076, 1.000000000000000000, 0.8660254037844387076, 1.000000000000000000, 0.8660254037844387076, 1.000000000000000000, 0.8660254037844387076, 1.000000000000000000, 0.8660254037844387076, 1.000000000000000000, 0.8660254037844387076, 1.000000000000000000, 0.8660254037844387076, 1.000000000000000000, 0.8660254037844387076, 1.000000000000000000, 0.8660254037844387076, 1.000000000000000000, 0.8660254037844387076, 1.000000000000000000, 0.8660254037844387076, 1.000000000000000000, 0.8660254037844387076, 1.000000000000000000, 0.8660254037844387076, 1.000000000000000000, 0.8660254037844387076, 1.000000000000000000, 0.8660254037844387076, 1.000000000000000000, 0.8660254037844387076, 1.000000000000000000, 0.8660254037844387076, 1.000000000000000000, 0.8660254037844387076, 1.000000000000000000, 0.8660254037844387076, 1.000000000000000000, 0.8660254037844387076, 1.000000000000000000, 0.8660254037844387076, 1.000000000000000000, 0.8660254037844387076, 1.000000000000000000, 0.8660254037844387076, 1.000000000000000000, 0.8660254037844387076, 1.000000000000000000, 0.8660254037844387076, 1.000000000000000000, 0.8660254037844387076, 1.000000000000000000, 0.8660254037844387076, 1.000000000000000000, 0.8660254037844387076, 1.000000000000000000, 0.8660254037844387076, 1.000000000000000000, 0.8660254037844387076, 1.000000000000000000, 0.8660254037844387076, 1.000000000000000000, 0.8660254037844387076, 1.000000000000000000, 0.8660254037844387076, 1.000000000000000000, 0.8660254037844387076, 1.000000000000000000, 0.8660254037844387076, 1.000000000000000000, 0.8660254037844387076, 1.000000000000000000, 0.8660254037844387076, 1.000000000000000000, 0.8660254037844387076, 1.000000000000000000, 0.8660254037844387076, 1.000000000000000000, 0.9111410770381633828, 0.9401538762233125901),
 ( 1.000000000000000000, 1.000000000000000000, 1.000000000000000000, 0.8660254037844387076, 1.000000000000000000, 0.8660254037844387076, 1.000000000000000000, 0.8660254037844387076, 1.000000000000000000, 0.8660254037844387076, 1.000000000000000000, 0.8660254037844387076, 1.000000000000000000, 0.8660254037844387076, 1.000000000000000000, 0.8660254037844387076, 1.000000000000000000, 0.8660254037844387076, 1.000000000000000000, 0.8660254037844387076, 1.000000000000000000, 0.8660254037844387076, 1.000000000000000000, 0.8660254037844387076, 1.000000000000000000, 0.8660254037844387076, 1.000000000000000000, 0.8660254037844387076, 1.000000000000000000, 0.8660254037844387076, 1.000000000000000000, 0.8660254037844387076, 1.000000000000000000, 0.8660254037844387076, 1.000000000000000000, 0.8660254037844387076, 1.000000000000000000, 0.8660254037844387076, 1.000000000000000000, 0.8660254037844387076, 1.000000000000000000, 0.8660254037844387076, 1.000000000000000000, 0.8660254037844387076, 1.000000000000000000, 0.8660254037844387076, 1.000000000000000000, 0.8660254037844387076, 1.000000000000000000, 0.8660254037844387076, 1.000000000000000000, 0.8660254037844387076, 1.000000000000000000, 0.8660254037844387076, 1.000000000000000000, 0.8660254037844387076, 1.000000000000000000, 0.8660254037844387076, 1.000000000000000000, 0.8660254037844387076, 1.000000000000000000, 0.8660254037844387076, 1.000000000000000000, 0.8660254037844387076, 1.000000000000000000, 0.8660254037844387076, 1.000000000000000000, 0.8660254037844387076, 1.000000000000000000, 0.8660254037844387076, 1.000000000000000000, 0.8660254037844387076, 1.000000000000000000, 0.8660254037844387076, 1.000000000000000000, 0.8660254037844387076, 1.000000000000000000, 0.8660254037844387076, 1.000000000000000000, 0.8660254037844387076, 1.000000000000000000, 0.8660254037844387076, 1.000000000000000000, 0.8660254037844387076, 1.000000000000000000, 0.8660254037844387076, 1.000000000000000000, 0.8660254037844387076, 1.000000000000000000, 0.8660254037844387076, 1.000000000000000000, 0.8660254037844387076, 1.000000000000000000, 0.8660254037844387076, 1.000000000000000000, 0.8660254037844387076, 1.000000000000000000, 0.8660254037844387076, 1.000000000000000000, 0.8660254037844387076, 1.000000000000000000, 0.8660254037844387076, 1.000000000000000000, 0.8660254037844387076, 1.000000000000000000, 0.8660254037844387076, 1.000000000000000000, 0.8660254037844387076, 1.000000000000000000, 0.8660254037844387076, 1.000000000000000000, 0.8660254037844387076, 1.000000000000000000, 0.8660254037844387076, 1.000000000000000000, 0.8660254037844387076, 1.000000000000000000, 0.8660254037844387076, 1.000000000000000000, 0.8660254037844387076, 1.000000000000000000, 0.8660254037844387076, 1.000000000000000000, 0.8660254037844387076, 1.000000000000000000, 0.8660254037844387076, 1.000000000000000000, 0.8660254037844387076, 1.000000000000000000, 0.8660254037844387076, 1.000000000000000000, 0.8660254037844387076, 1.000000000000000000, 0.8660254037844387076, 1.000000000000000000, 0.9111410770381633828, 0.9401538762233125901),
 ( 1.000000000000000000, 1.000000000000000000, 1.000000000000000000, 0.8660254037844387076, 1.000000000000000000, 0.8660254037844387076, 1.000000000000000000, 0.8660254037844387076, 1.000000000000000000, 0.8660254037844387076, 1.000000000000000000, 0.8660254037844387076, 1.000000000000000000, 0.8660254037844387076, 1.000000000000000000, 0.8660254037844387076, 1.000000000000000000, 0.8660254037844387076, 1.000000000000000000, 0.8660254037844387076, 1.000000000000000000, 0.8660254037844387076, 1.000000000000000000, 0.8660254037844387076, 1.000000000000000000, 0.8660254037844387076, 1.000000000000000000, 0.8660254037844387076, 1.000000000000000000, 0.8660254037844387076, 1.000000000000000000, 0.8660254037844387076, 1.000000000000000000, 0.8660254037844387076, 1.000000000000000000, 0.8660254037844387076, 1.000000000000000000, 0.8660254037844387076, 1.000000000000000000, 0.8660254037844387076, 1.000000000000000000, 0.8660254037844387076, 1.000000000000000000, 0.8660254037844387076, 1.000000000000000000, 0.8660254037844387076, 1.000000000000000000, 0.8660254037844387076, 1.000000000000000000, 0.8660254037844387076, 1.000000000000000000, 0.8660254037844387076, 1.000000000000000000, 0.8660254037844387076, 1.000000000000000000, 0.8660254037844387076, 1.000000000000000000, 0.8660254037844387076, 1.000000000000000000, 0.8660254037844387076, 1.000000000000000000, 0.8660254037844387076, 1.000000000000000000, 0.8660254037844387076, 1.000000000000000000, 0.8660254037844387076, 1.000000000000000000, 0.8660254037844387076, 1.000000000000000000, 0.8660254037844387076, 1.000000000000000000, 0.8660254037844387076, 1.000000000000000000, 0.8660254037844387076, 1.000000000000000000, 0.8660254037844387076, 1.000000000000000000, 0.8660254037844387076, 1.000000000000000000, 0.8660254037844387076, 1.000000000000000000, 0.8660254037844387076, 1.000000000000000000, 0.8660254037844387076, 1.000000000000000000, 0.8660254037844387076, 1.000000000000000000, 0.8660254037844387076, 1.000000000000000000, 0.8660254037844387076, 1.000000000000000000, 0.8660254037844387076, 1.000000000000000000, 0.8660254037844387076, 1.000000000000000000, 0.8660254037844387076, 1.000000000000000000, 0.8660254037844387076, 1.000000000000000000, 0.8660254037844387076, 1.000000000000000000, 0.8660254037844387076, 1.000000000000000000, 0.8660254037844387076, 1.000000000000000000, 0.8660254037844387076, 1.000000000000000000, 0.8660254037844387076, 1.000000000000000000, 0.8660254037844387076, 1.000000000000000000, 0.8660254037844387076, 1.000000000000000000, 0.8660254037844387076, 1.000000000000000000, 0.8660254037844387076, 1.000000000000000000, 0.8660254037844387076, 1.000000000000000000, 0.8660254037844387076, 1.000000000000000000, 0.8660254037844387076, 1.000000000000000000, 0.8660254037844387076, 1.000000000000000000, 0.8660254037844387076, 1.000000000000000000, 0.8660254037844387076, 1.000000000000000000, 0.8660254037844387076, 1.000000000000000000, 0.8660254037844387076, 1.000000000000000000, 0.8660254037844387076, 1.000000000000000000, 0.9111410770381633828, 0.9401538762233125901),
 ( 1.000000000000000000, 1.000000000000000000, 1.000000000000000000, 0.8660254037844387076, 1.000000000000000000, 0.8660254037844387076, 1.000000000000000000, 0.8660254037844387076, 1.000000000000000000, 0.8660254037844387076, 1.000000000000000000, 0.8660254037844387076, 1.000000000000000000, 0.8660254037844387076, 1.000000000000000000, 0.8660254037844387076, 1.000000000000000000, 0.8660254037844387076, 1.000000000000000000, 0.8660254037844387076, 1.000000000000000000, 0.8660254037844387076, 1.000000000000000000, 0.8660254037844387076, 1.000000000000000000, 0.8660254037844387076, 1.000000000000000000, 0.8660254037844387076, 1.000000000000000000, 0.8660254037844387076, 1.000000000000000000, 0.8660254037844387076, 1.000000000000000000, 0.8660254037844387076, 1.000000000000000000, 0.8660254037844387076, 1.000000000000000000, 0.8660254037844387076, 1.000000000000000000, 0.8660254037844387076, 1.000000000000000000, 0.8660254037844387076, 1.000000000000000000, 0.8660254037844387076, 1.000000000000000000, 0.8660254037844387076, 1.000000000000000000, 0.8660254037844387076, 1.000000000000000000, 0.8660254037844387076, 1.000000000000000000, 0.8660254037844387076, 1.000000000000000000, 0.8660254037844387076, 1.000000000000000000, 0.8660254037844387076, 1.000000000000000000, 0.8660254037844387076, 1.000000000000000000, 0.8660254037844387076, 1.000000000000000000, 0.8660254037844387076, 1.000000000000000000, 0.8660254037844387076, 1.000000000000000000, 0.8660254037844387076, 1.000000000000000000, 0.8660254037844387076, 1.000000000000000000, 0.8660254037844387076, 1.000000000000000000, 0.8660254037844387076, 1.000000000000000000, 0.8660254037844387076, 1.000000000000000000, 0.8660254037844387076, 1.000000000000000000, 0.8660254037844387076, 1.000000000000000000, 0.8660254037844387076, 1.000000000000000000, 0.8660254037844387076, 1.000000000000000000, 0.8660254037844387076, 1.000000000000000000, 0.8660254037844387076, 1.000000000000000000, 0.8660254037844387076, 1.000000000000000000, 0.8660254037844387076, 1.000000000000000000, 0.8660254037844387076, 1.000000000000000000, 0.8660254037844387076, 1.000000000000000000, 0.8660254037844387076, 1.000000000000000000, 0.8660254037844387076, 1.000000000000000000, 0.8660254037844387076, 1.000000000000000000, 0.8660254037844387076, 1.000000000000000000, 0.8660254037844387076, 1.000000000000000000, 0.8660254037844387076, 1.000000000000000000, 0.8660254037844387076, 1.000000000000000000, 0.8660254037844387076, 1.000000000000000000, 0.8660254037844387076, 1.000000000000000000, 0.8660254037844387076, 1.000000000000000000, 0.8660254037844387076, 1.000000000000000000, 0.8660254037844387076, 1.000000000000000000, 0.8660254037844387076, 1.000000000000000000, 0.8660254037844387076, 1.000000000000000000, 0.8660254037844387076, 1.000000000000000000, 0.8660254037844387076, 1.000000000000000000, 0.8660254037844387076, 1.000000000000000000, 0.8660254037844387076, 1.000000000000000000, 0.8660254037844387076, 1.000000000000000000, 0.8660254037844387076, 1.000000000000000000, 0.9111410770381633828, 0.9401538762233125901) ) ) 
 REPRESENTATION_ITEM ( '' )  SURFACE ( )  );
#12057=VERTEX_POINT ( 'NONE', #15585 ) ;
#12058=CARTESIAN_POINT ( 'NONE',  ( -85.39923668279692492, -34.99824194014708922, 99.66573144631155401 ) ) ;
#12063=CARTESIAN_POINT ( 'NONE',  ( -85.40000000000000568, -32.69606250001229597, 99.99999999999998579 ) ) ;
#12089=CARTESIAN_POINT ( 'NONE',  ( -83.90000000000000568, -32.72268749875867400, 97.40192378864668399 ) ) ;
#12091=CARTESIAN_POINT ( 'NONE',  ( -83.77821517812500929, -32.57812499938548711, 97.61286128772489690 ) ) ;
#12095=DIRECTION ( 'NONE',  ( -0.000000000000000000, -1.000000000000000000, -0.000000000000000000 ) ) ;
#12105=CARTESIAN_POINT ( 'NONE',  ( -82.39999999999999147, -32.95312499938548711, 96.81714838363319586 ) ) ;
#12110=CARTESIAN_POINT ( 'NONE',  ( -80.90000000000000568, -34.14374999877097139, 97.40192378864668399 ) ) ;
#12118=CARTESIAN_POINT ( 'NONE',  ( -85.40000000000000568, -30.37210047261201851, 100.9999487804559664 ) ) ;
#12120=CARTESIAN_POINT ( 'NONE',  ( -83.90000000000000568, -31.66874999877096997, 102.5980762113533018 ) ) ;
#12131=DIRECTION ( 'NONE',  ( -0.000000000000000000, -1.000000000000000000, -0.000000000000000000 ) ) ;
#12140=CARTESIAN_POINT ( 'NONE',  ( -82.39999999999999147, -31.68750000000000355, 103.4641016151377499 ) ) ;
#12145=( BOUNDED_CURVE ( )  B_SPLINE_CURVE ( 2, ( #5447, #8451, #12558, #3672, #15982, #9638, #950, #8167, #6708 ),
 .UNSPECIFIED., .F., .F. ) 
 B_SPLINE_CURVE_WITH_KNOTS ( ( 3, 2, 2, 2, 3 ),
 ( 0.2291666666666666297, 0.2361111111111111049, 0.2500000000000000000, 0.2638888888888888951, 0.2708333333333333148 ),
 .UNSPECIFIED. ) 
 CURVE ( )  GEOMETRIC_REPRESENTATION_ITEM ( )  RATIONAL_B_SPLINE_CURVE ( ( 0.9330127018922194093, 0.9330127018922190762, 1.000000000000000000, 0.8660254037844387076, 1.000000000000000000, 0.8660254037844387076, 1.000000000000000000, 0.9330127018922196314, 0.9330127018922194093 ) ) 
 REPRESENTATION_ITEM ( '' )  );
#12152=CARTESIAN_POINT ( 'NONE',  ( -81.59615242270662350, -31.61115380933863506, 102.9999999999999858 ) ) ;
#12155=CARTESIAN_POINT ( 'NONE',  ( -81.02178482187500208, -31.75312499938548427, 97.61286128772489690 ) ) ;
#12159=CARTESIAN_POINT ( 'NONE',  ( -79.96926199426660276, -35.00059217315788374, 101.7920197322231104 ) ) ;
#12162=CARTESIAN_POINT ( 'NONE',  ( -79.39999999999999147, -30.67500000000000071, 99.99999999999998579 ) ) ;
#12164=CARTESIAN_POINT ( 'NONE',  ( -85.15643035625001289, -30.29062499938548569, 98.40857419181659793 ) ) ;
#12165=CARTESIAN_POINT ( 'NONE',  ( -79.39999999999999147, -32.88750000000000284, 98.26794919243110371 ) ) ;
#12185=CARTESIAN_POINT ( 'NONE',  ( -85.40000000000000568, -31.78518749875867400, 98.26794919243111792 ) ) ;
#12203=CARTESIAN_POINT ( 'NONE',  ( -79.39999999999999147, -34.21874999877096712, 99.99999999999998579 ) ) ;
#12209=CARTESIAN_POINT ( 'NONE',  ( -81.59615242270662350, -34.36740381056766580, 102.9999999999999858 ) ) ;
#12210=CARTESIAN_POINT ( 'NONE',  ( -83.90000000000000568, -30.46874999877096712, 97.40192378864668399 ) ) ;
#12211=CARTESIAN_POINT ( 'NONE',  ( -85.40000000000000568, -32.15624999877096712, 101.7320508075688679 ) ) ;
#12213=ADVANCED_FACE ( 'NONE', ( #8025 ), #6769, .T. ) ;
#12250=CARTESIAN_POINT ( 'NONE',  ( -85.15643035624999868, -30.66562499938548569, 101.5914258081833879 ) ) ;
#12254=CARTESIAN_POINT ( 'NONE',  ( -80.42875664086302834, -34.99897389098457978, 97.71408729985186881 ) ) ;
#12261=EDGE_CURVE ( 'NONE', #17075, #1272, #5335, .T. ) ;
#12263=CARTESIAN_POINT ( 'NONE',  ( -85.15643035625001289, -31.15312499938548996, 99.99999999999998579 ) ) ;
#12278=ORIENTED_EDGE ( 'NONE', *, *, #3028, .T. ) ;
#12285=CARTESIAN_POINT ( 'NONE',  ( -79.39999999999999147, -34.18518749875867258, 98.26794919243110371 ) ) ;
#12299=CARTESIAN_POINT ( 'NONE',  ( -82.39999999999999147, -34.97812499938548569, 103.1828516163667899 ) ) ;
#12301=EDGE_LOOP ( 'NONE', ( #15116, #3247, #112 ) ) ;
#12306=CARTESIAN_POINT ( 'NONE',  ( -85.40000000000000568, -31.29374999877096997, 99.99999999999998579 ) ) ;
#12308=CARTESIAN_POINT ( 'NONE',  ( -82.40000000000000568, -30.00000000000000355, 96.99999999999998579 ) ) ;
#12309=CARTESIAN_POINT ( 'NONE',  ( -82.39999999999999147, -30.73124999877096641, 103.4641016151377499 ) ) ;
#12310=CARTESIAN_POINT ( 'NONE',  ( -85.40000000000000568, -34.89374999877097139, 99.99999999999998579 ) ) ;
#12328=ORIENTED_EDGE ( 'NONE', *, *, #5910, .F. ) ;
#12347=CARTESIAN_POINT ( 'NONE',  ( -79.64356964375001269, -30.96562499938548640, 101.5914258081833879 ) ) ;
#12352=CARTESIAN_POINT ( 'NONE',  ( -80.84132516849733463, -34.99999918353109507, 97.43127812267456989 ) ) ;
#12356=CARTESIAN_POINT ( 'NONE',  ( -82.39999999999999147, -30.36562499938548854, 96.81714838363319586 ) ) ;
#12380=CARTESIAN_POINT ( 'NONE',  ( -79.39999999999999147, -33.77268749875867826, 99.99999999999998579 ) ) ;
#12385=CARTESIAN_POINT ( 'NONE',  ( -82.39999999999999147, -31.23750000000000071, 102.9999999999999858 ) ) ;
#12393=CARTESIAN_POINT ( 'NONE',  ( -83.77821517812500929, -33.81562499938548427, 97.61286128772489690 ) ) ;
#12396=VERTEX_POINT ( 'NONE', #10273 ) ;
#12405=CARTESIAN_POINT ( 'NONE',  ( -83.90000000000000568, -33.01874999877097139, 102.5980762113533018 ) ) ;
#12406=CARTESIAN_POINT ( 'NONE',  ( -82.39999999999999147, -34.10624999877096997, 96.53589838486223584 ) ) ;
#12408=CARTESIAN_POINT ( 'NONE',  ( -79.39999999999999147, -30.65624999877096712, 101.7320508075688537 ) ) ;
#12420=ORIENTED_EDGE ( 'NONE', *, *, #5720, .F. ) ;
#12441=CARTESIAN_POINT ( 'NONE',  ( -85.15643035624999868, -32.01562499938548711, 101.5914258081833879 ) ) ;
#12444=ORIENTED_EDGE ( 'NONE', *, *, #5654, .T. ) ;
#12450=CARTESIAN_POINT ( 'NONE',  ( -82.39999999999999147, -32.61562499938548854, 96.81714838363319586 ) ) ;
#12465=PRODUCT ( 'leg', 'leg', '', ( #15418 ) ) ;
#12468=CARTESIAN_POINT ( 'NONE',  ( -85.40000000000000568, -30.03749999999999787, 98.26794919243111792 ) ) ;
#12472=CARTESIAN_POINT ( 'NONE',  ( -82.39999999999999147, -35.01018749875868252, 96.53589838486223584 ) ) ;
#12474=CARTESIAN_POINT ( 'NONE',  ( -82.39999999999999147, -34.86562499938548854, 96.81714838363319586 ) ) ;
#12485=CARTESIAN_POINT ( 'NONE',  ( -82.39999999999999147, -32.27812499938548285, 103.1828516163667899 ) ) ;
#12493=CARTESIAN_POINT ( 'NONE',  ( -82.39999999999999147, -31.40624999877096712, 96.99999999999998579 ) ) ;
#12495=CARTESIAN_POINT ( 'NONE',  ( -79.39999999999999147, -33.86250000000000426, 101.7320508075688537 ) ) ;
#12496=CARTESIAN_POINT ( 'NONE',  ( -85.40000000000000568, -31.29374999877096997, 99.99999999999998579 ) ) ;
#12498=CARTESIAN_POINT ( 'NONE',  ( -82.39999999999999147, -33.88124999877096855, 103.4641016151377499 ) ) ;
#12507=PRODUCT_DEFINITION ( 'UNKNOWN', '', #15500, #4759 ) ;
#12511=UNCERTAINTY_MEASURE_WITH_UNIT (LENGTH_MEASURE( 1.000000000000000082E-05 ), #15251, 'distance_accuracy_value', 'NONE');
#12513=ORIENTED_EDGE ( 'NONE', *, *, #13417, .T. ) ;
#12516=VERTEX_POINT ( 'NONE', #15043 ) ;
#12517=CARTESIAN_POINT ( 'NONE',  ( -82.40000000000001990, -31.18124999877096926, 103.0000000000000000 ) ) ;
#12521=CARTESIAN_POINT ( 'NONE',  ( -79.39999999999999147, -34.68356250001230023, 98.26794919243110371 ) ) ;
#12532=CARTESIAN_POINT ( 'NONE',  ( -83.20384757729335945, -33.90134618820329848, 102.9999999999999716 ) ) ;
#12534=CARTESIAN_POINT ( 'NONE',  ( -81.02178482187500208, -31.45312499938549067, 102.3871387122750889 ) ) ;
#12539=CARTESIAN_POINT ( 'NONE',  ( -79.39999999999999147, -34.70624999877097139, 101.7320508075688537 ) ) ;
#12544=CARTESIAN_POINT ( 'NONE',  ( -82.39999999999999147, -31.49062499938548143, 103.1828516163667899 ) ) ;
#12554=VECTOR ( 'NONE', #16903, 1000.000000000000000 ) ;
#12558=CARTESIAN_POINT ( 'NONE',  ( -83.90000000000000568, -31.27500000000000568, 102.5980762113533018 ) ) ;
#12567=CARTESIAN_POINT ( 'NONE',  ( -85.40000000000000568, -33.54768749875866973, 99.99999999999998579 ) ) ;
#12568=VERTEX_POINT ( 'NONE', #14950 ) ;
#12583=CARTESIAN_POINT ( 'NONE',  ( -85.15643035625001289, -34.64062499938548711, 99.99999999999998579 ) ) ;
#12593=CARTESIAN_POINT ( 'NONE',  ( -81.59615242270663771, -32.11740381056766580, 103.0000000000000000 ) ) ;
#12594=CARTESIAN_POINT ( 'NONE',  ( -85.40000000000000568, -31.78124999877096712, 98.26794919243111792 ) ) ;
#12595=CARTESIAN_POINT ( 'NONE',  ( -80.90000000000000568, -32.94374999877096855, 102.5980762113533018 ) ) ;
#12597=( BOUNDED_CURVE ( )  B_SPLINE_CURVE ( 2, ( #3734, #17513, #12917, #1095, #9699, #3929, #12822, #2465, #18787 ),
 .UNSPECIFIED., .F., .F. ) 
 B_SPLINE_CURVE_WITH_KNOTS ( ( 3, 2, 2, 2, 3 ),
 ( 0.1875000000000000000, 0.1944444444444444475, 0.2083333333333333426, 0.2222222222222222099, 0.2291666666666666297 ),
 .UNSPECIFIED. ) 
 CURVE ( )  GEOMETRIC_REPRESENTATION_ITEM ( )  RATIONAL_B_SPLINE_CURVE ( ( 0.9330127018922194093, 0.9330127018922194093, 1.000000000000000000, 0.8660254037844387076, 1.000000000000000000, 0.8660254037844387076, 1.000000000000000000, 0.9330127018922196314, 0.9330127018922194093 ) ) 
 REPRESENTATION_ITEM ( '' )  );
#12601=ORIENTED_EDGE ( 'NONE', *, *, #14734, .F. ) ;
#12608=FACE_OUTER_BOUND ( 'NONE', #3743, .T. ) ;
#12617=CARTESIAN_POINT ( 'NONE',  ( -85.40000000000000568, -34.04606250001229739, 99.99999999999998579 ) ) ;
#12622=CARTESIAN_POINT ( 'NONE',  ( -82.39999999999999147, -33.48750000000000426, 103.0000000000000000 ) ) ;
#12629=CARTESIAN_POINT ( 'NONE',  ( -85.40000000000000568, -33.95624999877097139, 101.7320508075688821 ) ) ;
#12631=CARTESIAN_POINT ( 'NONE',  ( -85.15643035625001289, -34.75312499938548427, 99.99999999999998579 ) ) ;
#12640=CARTESIAN_POINT ( 'NONE',  ( -82.39999999999999147, -33.29062499938548569, 103.1828516163667899 ) ) ;
#12650=CARTESIAN_POINT ( 'NONE',  ( -85.40000000000000568, -33.09374999877096712, 99.99999999999998579 ) ) ;
#12651=CARTESIAN_POINT ( 'NONE',  ( -83.90000000000000568, -34.12500000000000000, 97.40192378864668399 ) ) ;
#12659=CARTESIAN_POINT ( 'NONE',  ( -82.39999999999999147, -32.98124999877096286, 102.9999999999999858 ) ) ;
#12661=CARTESIAN_POINT ( 'NONE',  ( -80.90000000000000568, -33.84768749875867400, 102.5980762113533018 ) ) ;
#12670=( BOUNDED_CURVE ( )  B_SPLINE_CURVE ( 2, ( #11095, #3679, #16874, #2014, #8173, #9644, #15605, #6713, #12659 ),
 .UNSPECIFIED., .F., .F. ) 
 B_SPLINE_CURVE_WITH_KNOTS ( ( 3, 2, 2, 2, 3 ),
 ( 0.4374999999999999445, 0.4444444444444444198, 0.4583333333333333148, 0.4722222222222222099, 0.4791666666666666297 ),
 .UNSPECIFIED. ) 
 CURVE ( )  GEOMETRIC_REPRESENTATION_ITEM ( )  RATIONAL_B_SPLINE_CURVE ( ( 0.9330127018922192983, 0.9330127018922187432, 1.000000000000000000, 0.8660254037844387076, 1.000000000000000000, 0.8660254037844387076, 1.000000000000000000, 0.9330127018922196314, 0.9330127018922194093 ) ) 
 REPRESENTATION_ITEM ( '' )  );
#12677=CARTESIAN_POINT ( 'NONE',  ( -85.15643035624999868, -33.25312499938548427, 101.5914258081833879 ) ) ;
#12683=EDGE_LOOP ( 'NONE', ( #16226, #1254, #7852, #16074 ) ) ;
#12690=CARTESIAN_POINT ( 'NONE',  ( -79.39999999999999147, -33.28124999877096712, 98.26794919243110371 ) ) ;
#12691=CARTESIAN_POINT ( 'NONE',  ( -85.40000000000000568, -34.44374999877096855, 99.99999999999998579 ) ) ;
#12694=CARTESIAN_POINT ( 'NONE',  ( -82.40000000000000568, -33.71249999999998437, 96.99999999999998579 ) ) ;
#12704=CARTESIAN_POINT ( 'NONE',  ( -81.02178482187500208, -31.34062499938548996, 102.3871387122750889 ) ) ;
#12705=AXIS2_PLACEMENT_3D ( 'NONE', #17106, #3717, #9682 ) ;
#12707=ORIENTED_EDGE ( 'NONE', *, *, #9854, .F. ) ;
#12720=CARTESIAN_POINT ( 'NONE',  ( -80.90000000000000568, -34.64606250001229171, 97.40192378864668399 ) ) ;
#12732=AXIS2_PLACEMENT_3D ( 'NONE', #10563, #9281, #10749 ) ;
#12735=CARTESIAN_POINT ( 'NONE',  ( -83.77821517812500929, -34.22812499938549280, 102.3871387122750889 ) ) ;
#12740=CARTESIAN_POINT ( 'NONE',  ( -83.77821517812500929, -34.71562499938548285, 97.61286128772489690 ) ) ;
#12741=CARTESIAN_POINT ( 'NONE',  ( -80.90000000000000568, -34.59374999877096712, 97.40192378864668399 ) ) ;
#12746=CARTESIAN_POINT ( 'NONE',  ( -79.64356964374998427, -33.14062499938548711, 98.40857419181659793 ) ) ;
#12752=ORIENTED_EDGE ( 'NONE', *, *, #555, .F. ) ;
#12755=CARTESIAN_POINT ( 'NONE',  ( -85.40000000000000568, -34.05000000000000426, 99.99999999999998579 ) ) ;
#12763=CARTESIAN_POINT ( 'NONE',  ( -83.90000000000000568, -30.07499999999999929, 97.40192378864668399 ) ) ;
#12764=CARTESIAN_POINT ( 'NONE',  ( -83.90000000000000568, -30.07106250001229242, 97.40192378864668399 ) ) ;
#12765=DIRECTION ( 'NONE',  ( -0.000000000000000000, -1.000000000000000000, -0.000000000000000000 ) ) ;
#12780=CARTESIAN_POINT ( 'NONE',  ( -83.77821517812500929, -32.46562499938548285, 97.61286128772489690 ) ) ;
#12790=CARTESIAN_POINT ( 'NONE',  ( -83.90000000000000568, -31.81874999877096855, 97.40192378864668399 ) ) ;
#12791=CARTESIAN_POINT ( 'NONE',  ( -82.39999999999999147, -31.71562499938548640, 96.81714838363319586 ) ) ;
#12794=DIRECTION ( 'NONE',  ( -0.000000000000000000, -1.000000000000000000, -0.000000000000000000 ) ) ;
#12803=CARTESIAN_POINT ( 'NONE',  ( -85.40000000000000568, -35.34374999877096712, 99.99999999999998579 ) ) ;
#12804=CARTESIAN_POINT ( 'NONE',  ( -82.39999999999999147, -30.25312499938548783, 96.81714838363319586 ) ) ;
#12809=ORIENTED_EDGE ( 'NONE', *, *, #3608, .F. ) ;
#12816=CARTESIAN_POINT ( 'NONE',  ( -82.39999999999999147, -34.60856250001229739, 96.53589838486223584 ) ) ;
#12817=CARTESIAN_POINT ( 'NONE',  ( -85.40000000000000568, -30.39374999877097139, 99.99999999999998579 ) ) ;
#12818=DIRECTION ( 'NONE',  ( 0.000000000000000000, 0.000000000000000000, 1.000000000000000000 ) ) ;
#12822=CARTESIAN_POINT ( 'NONE',  ( -80.90000000000000568, -31.20000000000000284, 102.5980762113533018 ) ) ;
#12829=CARTESIAN_POINT ( 'NONE',  ( -82.39999999999999147, -33.51562499938548001, 96.81714838363319586 ) ) ;
#12835=CARTESIAN_POINT ( 'NONE',  ( -83.77821517812500929, -33.21562499938548285, 102.3871387122750889 ) ) ;
#12840=CARTESIAN_POINT ( 'NONE',  ( -81.02178482187500208, -34.60312499938549280, 102.3871387122750889 ) ) ;
#12850=CARTESIAN_POINT ( 'NONE',  ( -85.40000000000000568, -34.50000000000000000, 99.99999999999998579 ) ) ;
#12857=CARTESIAN_POINT ( 'NONE',  ( -82.40000000000000568, -30.00000000000000355, 103.0000000000000000 ) ) ;
#12859=CARTESIAN_POINT ( 'NONE',  ( -83.90000000000000568, -30.97106250001229100, 97.40192378864668399 ) ) ;
#12863=CARTESIAN_POINT ( 'NONE',  ( -83.77821517812500929, -30.66562499938548569, 97.61286128772489690 ) ) ;
#12864=CARTESIAN_POINT ( 'NONE',  ( -85.40000000000000568, -33.60000000000000142, 99.99999999999998579 ) ) ;
#12886=CARTESIAN_POINT ( 'NONE',  ( -80.90000000000000568, -35.19374999877096855, 102.5980762113533018 ) ) ;
#12887=CARTESIAN_POINT ( 'NONE',  ( -84.69813954184694182, -35.39427337414329600, 98.07164457472185859 ) ) ;
#12897=VERTEX_POINT ( 'NONE', #13740 ) ;
#12899=CARTESIAN_POINT ( 'NONE',  ( -85.40000000000000568, -35.36739040097838682, 98.90809659374339446 ) ) ;
#12901=CARTESIAN_POINT ( 'NONE',  ( -79.64356964374999848, -30.81562499938548427, 99.99999999999998579 ) ) ;
#12905=CARTESIAN_POINT ( 'NONE',  ( -82.40000000000000568, -33.65624999877097423, 97.00000000000000000 ) ) ;
#12906=VERTEX_POINT ( 'NONE', #11269 ) ;
#12911=CARTESIAN_POINT ( 'NONE',  ( -85.40000000000000568, -33.18750000000000000, 98.26794919243111792 ) ) ;
#12917=CARTESIAN_POINT ( 'NONE',  ( -80.90000000000000568, -31.05000000000000071, 97.40192378864668399 ) ) ;
#12920=CARTESIAN_POINT ( 'NONE',  ( -82.40000000000000568, -30.00000000000000355, 99.99999999999998579 ) ) ;
#12923=CARTESIAN_POINT ( 'NONE',  ( -81.02178482187500208, -32.80312499938548854, 102.3871387122750889 ) ) ;
#12926=CARTESIAN_POINT ( 'NONE',  ( -79.64356964375001269, -33.10312499938549280, 101.5914258081833879 ) ) ;
#12932=CARTESIAN_POINT ( 'NONE',  ( -85.15643035625001289, -34.79062499938548569, 98.40857419181659793 ) ) ;
#12943=CARTESIAN_POINT ( 'NONE',  ( -80.90000000000000568, -32.55000000000000426, 102.5980762113533018 ) ) ;
#12951=CARTESIAN_POINT ( 'NONE',  ( -82.40000000000000568, -30.00000000000000355, 103.0000000000000000 ) ) ;
#12956=CARTESIAN_POINT ( 'NONE',  ( -83.20384757729337366, -33.50759618943233420, 103.0000000000000000 ) ) ;
#12980=CARTESIAN_POINT ( 'NONE',  ( -79.39999999999999147, -34.25624999877096855, 101.7320508075688537 ) ) ;
#12981=CARTESIAN_POINT ( 'NONE',  ( -79.64356964375001269, -30.89062499938548711, 98.40857419181659793 ) ) ;
#13005=CARTESIAN_POINT ( 'NONE',  ( -85.40000000000000568, -32.21249999999999858, 101.7320508075688679 ) ) ;
#13006=CARTESIAN_POINT ( 'NONE',  ( -82.40000000000000568, -30.00000000000000355, 103.0000000000000000 ) ) ;
#13013=ORIENTED_EDGE ( 'NONE', *, *, #2950, .T. ) ;
#13019=CARTESIAN_POINT ( 'NONE',  ( -79.64356964374999848, -32.72812499938548569, 99.99999999999998579 ) ) ;
#13020=DIRECTION ( 'NONE',  ( 0.000000000000000000, -0.000000000000000000, -1.000000000000000000 ) ) ;
#13023=CARTESIAN_POINT ( 'NONE',  ( -83.77821517812500929, -34.11562499938548854, 102.3871387122750889 ) ) ;
#13029=CARTESIAN_POINT ( 'NONE',  ( -83.77821517812500929, -33.32812499938548711, 102.3871387122750889 ) ) ;
#13040=CARTESIAN_POINT ( 'NONE',  ( -85.40000000000000568, -33.11250000000000426, 101.7320508075688679 ) ) ;
#13050=CARTESIAN_POINT ( 'NONE',  ( -79.39999999999999147, -30.22106250001229100, 99.99999999999998579 ) ) ;
#13055=CARTESIAN_POINT ( 'NONE',  ( -82.40000000000000568, -33.71249999999998437, 96.99999999999998579 ) ) ;
#13062=VERTEX_POINT ( 'NONE', #1405 ) ;
#13076=CARTESIAN_POINT ( 'NONE',  ( -85.40000000000000568, -34.40624999877096712, 101.7320508075688679 ) ) ;
#13077=CARTESIAN_POINT ( 'NONE',  ( -85.15643035624999868, -32.01562499938548711, 101.5914258081833879 ) ) ;
#13088=CARTESIAN_POINT ( 'NONE',  ( -81.02178482187500208, -30.89062499938548711, 102.3871387122750889 ) ) ;
#13099=CARTESIAN_POINT ( 'NONE',  ( -83.90000000000000568, -32.32500000000000284, 97.40192378864668399 ) ) ;
#13102=CARTESIAN_POINT ( 'NONE',  ( -84.69814161231455785, -35.39427329483935836, 98.07164704222793716 ) ) ;
#13110=CARTESIAN_POINT ( 'NONE',  ( -85.15643035625001289, -30.14062499938548711, 99.99999999999998579 ) ) ;
#13111=FACE_OUTER_BOUND ( 'NONE', #14170, .T. ) ;
#13115=CARTESIAN_POINT ( 'NONE',  ( -82.39999999999999147, -34.07812499938548711, 103.1828516163667899 ) ) ;
#13139=CARTESIAN_POINT ( 'NONE',  ( -79.64356964374999848, -32.61562499938548854, 99.99999999999998579 ) ) ;
#13152=EDGE_CURVE ( 'NONE', #7760, #12057, #7350, .T. ) ;
#13165=CARTESIAN_POINT ( 'NONE',  ( -85.40000000000000568, -34.48124999877096997, 98.26794919243111792 ) ) ;
#13166=EDGE_CURVE ( 'NONE', #17250, #7672, #19089, .T. ) ;
#13167=CARTESIAN_POINT ( 'NONE',  ( -79.64356964375001269, -30.44062499938548783, 98.40857419181659793 ) ) ;
#13180=CARTESIAN_POINT ( 'NONE',  ( -82.39999999999999147, -32.27812499938548285, 103.1828516163667899 ) ) ;
#13193=CARTESIAN_POINT ( 'NONE',  ( -85.40000000000000568, -32.25000000000000000, 99.99999999999998579 ) ) ;
#13205=CARTESIAN_POINT ( 'NONE',  ( -81.02178482187500208, -30.74062499938548498, 97.61286128772489690 ) ) ;
#13206=CARTESIAN_POINT ( 'NONE',  ( -82.40000000000000568, -50.00000000000000000, 99.99999999999998579 ) ) ;
#13212=CARTESIAN_POINT ( 'NONE',  ( -79.39999999999999147, -30.22500000000000142, 99.99999999999998579 ) ) ;
#13218=CARTESIAN_POINT ( 'NONE',  ( -82.39999999999999147, -30.78750000000000142, 102.9999999999999858 ) ) ;
#13223=CARTESIAN_POINT ( 'NONE',  ( -80.90000000000000568, -31.44374999877096855, 97.40192378864668399 ) ) ;
#13227=CYLINDRICAL_SURFACE ( 'NONE', #2114, 7.500000000000020428 ) ;
#13235=CARTESIAN_POINT ( 'NONE',  ( -82.39999999999999147, -31.68356250001229313, 103.4641016151377499 ) ) ;
#13238=CARTESIAN_POINT ( 'NONE',  ( -82.39999999999999147, -32.72812499938548569, 103.1828516163667899 ) ) ;
#13239=CARTESIAN_POINT ( 'NONE',  ( -85.40000000000000568, -32.60624999877096997, 101.7320508075688821 ) ) ;
#13255=CARTESIAN_POINT ( 'NONE',  ( -82.40000000000001990, -32.75624999877096855, 97.00000000000000000 ) ) ;
#13257=CARTESIAN_POINT ( 'NONE',  ( -81.59615242270660929, -30.31740381056766509, 102.9999999999999858 ) ) ;
#13262=CARTESIAN_POINT ( 'NONE',  ( -82.39999999999999147, -34.10624999877096997, 96.53589838486223584 ) ) ;
#13263=CARTESIAN_POINT ( 'NONE',  ( -79.64356964375001269, -34.56562499938549138, 101.5914258081833879 ) ) ;
#13274=CARTESIAN_POINT ( 'NONE',  ( -83.77821517812500929, -32.76562499938548711, 102.3871387122750889 ) ) ;
#13282=CARTESIAN_POINT ( 'NONE',  ( -83.20384757729335945, -31.83615380933863648, 96.99999999999997158 ) ) ;
#13286=CARTESIAN_POINT ( 'NONE',  ( -85.40000000000000568, -33.14999999999999858, 99.99999999999998579 ) ) ;
#13287=CARTESIAN_POINT ( 'NONE',  ( -82.39999999999999147, -32.08124999877097139, 103.4641016151377499 ) ) ;
#13301=CARTESIAN_POINT ( 'NONE',  ( -79.64356964375001269, -31.22812499938548925, 98.40857419181659793 ) ) ;
#13302=CARTESIAN_POINT ( 'NONE',  ( -84.65149424414151724, -35.03567958137573868, 98.11078664818333550 ) ) ;
#13310=CARTESIAN_POINT ( 'NONE',  ( -79.39999999999999147, -31.98750000000000071, 98.26794919243110371 ) ) ;
#13314=CARTESIAN_POINT ( 'NONE',  ( -82.39999999999999147, -32.58750000000000568, 102.9999999999999858 ) ) ;
#13327=CARTESIAN_POINT ( 'NONE',  ( -84.69814068649969840, -35.00052333152936512, 98.07164593887567605 ) ) ;
#13334=CARTESIAN_POINT ( 'NONE',  ( -79.39999999999999147, -32.92106250001229739, 99.99999999999998579 ) ) ;
#13340=CARTESIAN_POINT ( 'NONE',  ( -85.15643035624999868, -32.35312499938549280, 101.5914258081833879 ) ) ;
#13360=CARTESIAN_POINT ( 'NONE',  ( -85.40000000000000568, -32.15624999877096712, 101.7320508075688821 ) ) ;
#13366=CARTESIAN_POINT ( 'NONE',  ( -82.39999999999999147, -31.63518749875868252, 103.4641016151377499 ) ) ;
#13367=CARTESIAN_POINT ( 'NONE',  ( -81.02178482187500208, -33.55312499938548854, 97.61286128772489690 ) ) ;
#13378=CARTESIAN_POINT ( 'NONE',  ( -85.15643035625001289, -34.19062499938548427, 99.99999999999998579 ) ) ;
#13382=CARTESIAN_POINT ( 'NONE',  ( -83.90000000000000568, -34.87500000000000000, 102.5980762113533018 ) ) ;
#13388=CARTESIAN_POINT ( 'NONE',  ( -85.40000000000000568, -30.80624999877096926, 101.7320508075688679 ) ) ;
#13389=( BOUNDED_CURVE ( )  B_SPLINE_CURVE ( 1, ( #2946, #16533 ),
 .UNSPECIFIED., .F., .F. ) 
 B_SPLINE_CURVE_WITH_KNOTS ( ( 2, 2 ),
 ( 0.000000000000000000, 1.000000000000000000 ),
 .UNSPECIFIED. ) 
 CURVE ( )  GEOMETRIC_REPRESENTATION_ITEM ( )  RATIONAL_B_SPLINE_CURVE ( ( 0.9401539645359766606, 0.9401539645359766606 ) ) 
 REPRESENTATION_ITEM ( '' )  );
#13390=CARTESIAN_POINT ( 'NONE',  ( -79.39999999999999147, -30.65624999877096712, 101.7320508075688537 ) ) ;
#13392=CARTESIAN_POINT ( 'NONE',  ( -82.40000000000000568, -30.00000000000000355, 99.99999999999998579 ) ) ;
#13402=CARTESIAN_POINT ( 'NONE',  ( -81.02178482187500208, -32.24062499938548854, 102.3871387122750889 ) ) ;
#13410=CARTESIAN_POINT ( 'NONE',  ( -83.90000000000000568, -30.82500000000000284, 102.5980762113533018 ) ) ;
#13417=EDGE_CURVE ( 'NONE', #9315, #15126, #16836, .T. ) ;
#13427=CARTESIAN_POINT ( 'NONE',  ( -83.90000000000000568, -34.87500000000000000, 102.5980762113533018 ) ) ;
#13433=CARTESIAN_POINT ( 'NONE',  ( -83.90000000000000568, -33.07106250001229597, 102.5980762113533018 ) ) ;
#13436=CARTESIAN_POINT ( 'NONE',  ( -82.39999999999999147, -32.27812499938548285, 103.1828516163667899 ) ) ;
#13437=CARTESIAN_POINT ( 'NONE',  ( -80.90000000000000568, -33.00000000000000000, 102.5980762113533018 ) ) ;
#13458=CARTESIAN_POINT ( 'NONE',  ( -79.39999999999999147, -32.83518749875868536, 98.26794919243110371 ) ) ;
#13459=CARTESIAN_POINT ( 'NONE',  ( -85.15643035625001289, -32.95312499938548711, 99.99999999999998579 ) ) ;
#13466=EDGE_LOOP ( 'NONE', ( #9557, #6436, #10942, #7087 ) ) ;
#13470=CARTESIAN_POINT ( 'NONE',  ( -85.15643035625001289, -34.64062499938548711, 99.99999999999998579 ) ) ;
#13472=EDGE_LOOP ( 'NONE', ( #19127, #10738, #17138 ) ) ;
#13475=CARTESIAN_POINT ( 'NONE',  ( -79.39999999999999147, -34.18124999877097281, 98.26794919243110371 ) ) ;
#13481=CARTESIAN_POINT ( 'NONE',  ( -79.39999999999999147, -34.23750000000000426, 98.26794919243110371 ) ) ;
#13482=CARTESIAN_POINT ( 'NONE',  ( -83.90000000000000568, -32.56874999877096855, 102.5980762113533018 ) ) ;
#13496=CARTESIAN_POINT ( 'NONE',  ( -85.15643035624999868, -31.07812499938548356, 98.40857419181659793 ) ) ;
#13502=CARTESIAN_POINT ( 'NONE',  ( -79.39999999999999147, -30.67500000000000071, 99.99999999999998579 ) ) ;
#13508=( BOUNDED_CURVE ( )  B_SPLINE_CURVE ( 2, ( #4972, #10913, #16879, #5062, #3483, #3583, #10127, #11397, #17170 ),
 .UNSPECIFIED., .F., .F. ) 
 B_SPLINE_CURVE_WITH_KNOTS ( ( 3, 2, 2, 2, 3 ),
 ( 0.7291666666666666297, 0.7361111111111111605, 0.7500000000000000000, 0.7638888888888888395, 0.7708333333333331483 ),
 .UNSPECIFIED. ) 
 CURVE ( )  GEOMETRIC_REPRESENTATION_ITEM ( )  RATIONAL_B_SPLINE_CURVE ( ( 0.9330127018922192983, 0.9330127018922187432, 1.000000000000000000, 0.8660254037844387076, 1.000000000000000000, 0.8660254037844387076, 1.000000000000000000, 0.9330127018922209636, 0.9330127018922194093 ) ) 
 REPRESENTATION_ITEM ( '' )  );
#13518=CARTESIAN_POINT ( 'NONE',  ( -83.33080762004576059, -35.05289549976084373, 96.44210921874548603 ) ) ;
#13524=CARTESIAN_POINT ( 'NONE',  ( -83.90000000000000568, -32.32106250001229597, 97.40192378864668399 ) ) ;
#13535=FACE_OUTER_BOUND ( 'NONE', #7605, .T. ) ;
#13546=EDGE_CURVE ( 'NONE', #7994, #9630, #2436, .T. ) ;
#13549=CARTESIAN_POINT ( 'NONE',  ( -79.39999999999999147, -31.97268749875867400, 99.99999999999998579 ) ) ;
#13550=CARTESIAN_POINT ( 'NONE',  ( -85.15643035624999868, -33.44062499938548427, 98.40857419181659793 ) ) ;
#13553=CARTESIAN_POINT ( 'NONE',  ( -82.40000000000000568, -30.00000000000000355, 96.99999999999998579 ) ) ;
#13556=ORIENTED_EDGE ( 'NONE', *, *, #14832, .F. ) ;
#13562=CARTESIAN_POINT ( 'NONE',  ( -81.02178482187500208, -32.99062499938548854, 97.61286128772489690 ) ) ;
#13563=ORIENTED_EDGE ( 'NONE', *, *, #2937, .F. ) ;
#13564=ORIENTED_EDGE ( 'NONE', *, *, #1328, .T. ) ;
#13571=( GEOMETRIC_REPRESENTATION_CONTEXT ( 3 ) GLOBAL_UNCERTAINTY_ASSIGNED_CONTEXT ( ( #13588 ) ) GLOBAL_UNIT_ASSIGNED_CONTEXT ( ( #14363, #8315, #9689 ) ) REPRESENTATION_CONTEXT ( 'NONE', 'WORKASPACE' ) );
#13573=CARTESIAN_POINT ( 'NONE',  ( -85.40000000000000568, -34.50000000000000000, 99.99999999999998579 ) ) ;
#13575=CARTESIAN_POINT ( 'NONE',  ( -80.90000000000000568, -31.14374999877097139, 102.5980762113533018 ) ) ;
#13584=CARTESIAN_POINT ( 'NONE',  ( -82.40000000000000568, -30.00000000000000355, 99.99999999999998579 ) ) ;
#13588=UNCERTAINTY_MEASURE_WITH_UNIT (LENGTH_MEASURE( 1.000000000000000082E-05 ), #14363, 'distance_accuracy_value', 'NONE');
#13593=CARTESIAN_POINT ( 'NONE',  ( -85.40000000000000568, -30.90000000000000213, 99.99999999999998579 ) ) ;
#13608=CARTESIAN_POINT ( 'NONE',  ( -85.15643035624999868, -30.74062499938548143, 98.40857419181659793 ) ) ;
#13612=CARTESIAN_POINT ( 'NONE',  ( -82.67676497412369940, -35.00026477264749047, 103.0072806454569303 ) ) ;
#13616=CARTESIAN_POINT ( 'NONE',  ( -82.39999999999999147, -33.70856250001228460, 96.53589838486223584 ) ) ;
#13619=CARTESIAN_POINT ( 'NONE',  ( -79.64356964374999848, -30.47812499938548569, 99.99999999999998579 ) ) ;
#13633=DIRECTION ( 'NONE',  ( -0.000000000000000000, -1.000000000000000000, -0.000000000000000000 ) ) ;
#13634=EDGE_LOOP ( 'NONE', ( #7611, #1863, #3696, #6283 ) ) ;
#13645=CARTESIAN_POINT ( 'NONE',  ( -82.39999999999999147, -31.41018749875868110, 96.53589838486223584 ) ) ;
#13648=CARTESIAN_POINT ( 'NONE',  ( -81.02178482187500208, -33.10312499938548569, 97.61286128772489690 ) ) ;
#13671=ORIENTED_EDGE ( 'NONE', *, *, #7675, .F. ) ;
#13676=CARTESIAN_POINT ( 'NONE',  ( -85.40000000000000568, -30.43124999877096926, 98.26794919243111792 ) ) ;
#13677=CARTESIAN_POINT ( 'NONE',  ( -79.39999999999999147, -31.51874999877096784, 99.99999999999998579 ) ) ;
#13683=ORIENTED_EDGE ( 'NONE', *, *, #8266, .F. ) ;
#13688=EDGE_CURVE ( 'NONE', #6735, #7760, #19071, .T. ) ;
#13689=CARTESIAN_POINT ( 'NONE',  ( -83.20384757729338787, -33.63615380933863719, 97.00000000000000000 ) ) ;
#13712=CARTESIAN_POINT ( 'NONE',  ( -82.39999999999999147, -31.49062499938548854, 103.1828516163667899 ) ) ;
#13716=CARTESIAN_POINT ( 'NONE',  ( -79.60928765286361397, -35.00091442770696659, 98.84622810931887216 ) ) ;
#13720=CARTESIAN_POINT ( 'NONE',  ( -82.39999999999999147, -30.59062499938548640, 103.1828516163667899 ) ) ;
#13740=CARTESIAN_POINT ( 'NONE',  ( -82.40000000000000568, -35.00000000000000000, 92.49999999999997158 ) ) ;
#13742=CARTESIAN_POINT ( 'NONE',  ( -82.39999999999999147, -32.08518749875868536, 103.4641016151377499 ) ) ;
#13751=ADVANCED_FACE ( 'NONE', ( #4313 ), #6612, .T. ) ;
#13768=CARTESIAN_POINT ( 'NONE',  ( -80.90000000000000568, -33.89999999999999858, 102.5980762113533018 ) ) ;
#13769=CARTESIAN_POINT ( 'NONE',  ( -83.90000000000000568, -30.91874999877096997, 97.40192378864668399 ) ) ;
#13770=CARTESIAN_POINT ( 'NONE',  ( -85.40000000000000568, -34.85624999877096997, 101.7320508075688679 ) ) ;
#13771=CARTESIAN_POINT ( 'NONE',  ( -82.40000000000001990, -32.08124999877097139, 103.0000000000000000 ) ) ;
#13776=EDGE_CURVE ( 'NONE', #7903, #10919, #5061, .T. ) ;
#13788=ORIENTED_EDGE ( 'NONE', *, *, #10678, .F. ) ;
#13803=CARTESIAN_POINT ( 'NONE',  ( -83.77821517812500929, -32.12812499938548427, 97.61286128772489690 ) ) ;
#13808=CARTESIAN_POINT ( 'NONE',  ( -80.85786485831481230, -34.99991206035976887, 102.5785900675527813 ) ) ;
#13813=CARTESIAN_POINT ( 'NONE',  ( -85.15643035625001289, -32.50312499938548427, 99.99999999999998579 ) ) ;
#13833=CARTESIAN_POINT ( 'NONE',  ( -85.40000000000000568, -33.51018749875867542, 101.7320508075688679 ) ) ;
#13834=ORIENTED_EDGE ( 'NONE', *, *, #8150, .F. ) ;
#13842=ORIENTED_EDGE ( 'NONE', *, *, #10207, .T. ) ;
#13847=CARTESIAN_POINT ( 'NONE',  ( -85.15643035625001289, -33.74062499938548854, 99.99999999999998579 ) ) ;
#13857=CARTESIAN_POINT ( 'NONE',  ( -79.39999999999999147, -33.78750000000000853, 98.26794919243110371 ) ) ;
#13858=CARTESIAN_POINT ( 'NONE',  ( -85.40000000000000568, -32.15624999877096712, 101.7320508075688679 ) ) ;
#13859=CARTESIAN_POINT ( 'NONE',  ( -79.39999999999999147, -33.28124999877096712, 98.26794919243110371 ) ) ;
#13860=PRODUCT_DEFINITION_SHAPE ( 'NONE', 'NONE',  #12507 ) ;
#13866=PRESENTATION_STYLE_ASSIGNMENT (( #3131 ) ) ;
#13893=( BOUNDED_CURVE ( )  B_SPLINE_CURVE ( 2, ( #8617, #16340, #7251, #4228, #14865, #5791, #7446, #5700, #8715 ),
 .UNSPECIFIED., .F., .F. ) 
 B_SPLINE_CURVE_WITH_KNOTS ( ( 3, 2, 2, 2, 3 ),
 ( 0.7291666666666668517, 0.7361111111111111605, 0.7500000000000000000, 0.7638888888888888395, 0.7708333333333333703 ),
 .UNSPECIFIED. ) 
 CURVE ( )  GEOMETRIC_REPRESENTATION_ITEM ( )  RATIONAL_B_SPLINE_CURVE ( ( 0.9330127018922194093, 0.9330127018922209636, 1.000000000000000000, 0.8660254037844387076, 1.000000000000000000, 0.8660254037844387076, 1.000000000000000000, 0.9330127018922187432, 0.9330127018922192983 ) ) 
 REPRESENTATION_ITEM ( '' )  );
#13896=CARTESIAN_POINT ( 'NONE',  ( -85.40000000000000568, -30.93750000000000355, 98.26794919243111792 ) ) ;
#13898=CARTESIAN_POINT ( 'NONE',  ( -81.02178482187500208, -32.35312499938548569, 102.3871387122750889 ) ) ;
#13904=VECTOR ( 'NONE', #10027, 1000.000000000000000 ) ;
#13909=CARTESIAN_POINT ( 'NONE',  ( -85.15643035625001289, -32.46562499938548996, 101.5914258081833879 ) ) ;
#13924=CYLINDRICAL_SURFACE ( 'NONE', #8048, 3.000000000000002665 ) ;
#13928=DIRECTION ( 'NONE',  ( -0.000000000000000000, -1.000000000000000000, -0.000000000000000000 ) ) ;
#13932=CARTESIAN_POINT ( 'NONE',  ( -79.39999999999999147, -34.67268749875867684, 99.99999999999998579 ) ) ;
#13935=CARTESIAN_POINT ( 'NONE',  ( -85.15643035624999868, -35.16562499938547859, 101.5914258081833879 ) ) ;
#13936=DIRECTION ( 'NONE',  ( 0.000000000000000000, 0.000000000000000000, -1.000000000000000000 ) ) ;
#13949=CARTESIAN_POINT ( 'NONE',  ( -83.77821517812500929, -32.76562499938548711, 102.3871387122750889 ) ) ;
#13950=CARTESIAN_POINT ( 'NONE',  ( -79.64356964374998427, -34.82812499938548711, 98.40857419181659793 ) ) ;
#13954=DIRECTION ( 'NONE',  ( -0.000000000000000000, -1.000000000000000000, -0.000000000000000000 ) ) ;
#13959=CARTESIAN_POINT ( 'NONE',  ( -81.59615242270662350, -31.93259618943233846, 97.00000000000000000 ) ) ;
#13960=CARTESIAN_POINT ( 'NONE',  ( -79.39999999999999147, -31.03124999877097068, 98.26794919243110371 ) ) ;
#13961=CARTESIAN_POINT ( 'NONE',  ( -79.39999999999999147, -35.08124999877097139, 98.26794919243110371 ) ) ;
#13963=CARTESIAN_POINT ( 'NONE',  ( -79.39999999999999147, -30.58124999877097139, 98.26794919243110371 ) ) ;
#13985=DIRECTION ( 'NONE',  ( 0.000000000000000000, 0.000000000000000000, -1.000000000000000000 ) ) ;
#13987=CARTESIAN_POINT ( 'NONE',  ( -80.90000000000000568, -34.79606250001229739, 102.5980762113533018 ) ) ;
#13990=CARTESIAN_POINT ( 'NONE',  ( -80.90000000000000568, -33.45000000000000284, 102.5980762113533018 ) ) ;
#14000=CARTESIAN_POINT ( 'NONE',  ( -85.15643035624999868, -31.64062499938548356, 98.40857419181659793 ) ) ;
#14011=CARTESIAN_POINT ( 'NONE',  ( -81.02178482187500208, -31.75312499938548427, 97.61286128772489690 ) ) ;
#14030=DIRECTION ( 'NONE',  ( -0.000000000000000000, -1.000000000000000000, -0.000000000000000000 ) ) ;
#14033=CARTESIAN_POINT ( 'NONE',  ( -80.90000000000000568, -33.39768749875867826, 102.5980762113533018 ) ) ;
#14048=CARTESIAN_POINT ( 'NONE',  ( -82.39999999999999147, -34.52812499938548996, 103.1828516163667899 ) ) ;
#14049=CARTESIAN_POINT ( 'NONE',  ( -79.64356964374998427, -34.90312499938548285, 101.5914258081833879 ) ) ;
#14059=CARTESIAN_POINT ( 'NONE',  ( -81.59615242270662350, -34.18259618943233136, 96.99999999999998579 ) ) ;
#14060=CARTESIAN_POINT ( 'NONE',  ( -80.90000000000000568, -32.49374999877097281, 102.5980762113533018 ) ) ;
#14061=CARTESIAN_POINT ( 'NONE',  ( -85.40000000000000568, -33.54374999877096286, 99.99999999999998579 ) ) ;
#14068=SHAPE_REPRESENTATION_RELATIONSHIP ( 'NONE' , 'NONE' ,  #16991, #18578 ) ;
#14082=CARTESIAN_POINT ( 'NONE',  ( -79.39999999999999147, -30.26249999999999929, 101.7320508075688537 ) ) ;
#14094=CARTESIAN_POINT ( 'NONE',  ( -81.02178482187500208, -34.45312499938548711, 97.61286128772489690 ) ) ;
#14104=CARTESIAN_POINT ( 'NONE',  ( -79.64356964374999848, -33.62812499938548427, 99.99999999999998579 ) ) ;
#14124=CARTESIAN_POINT ( 'NONE',  ( -85.40000000000000568, -35.31018749875867258, 101.7320508075688679 ) ) ;
#14125=CARTESIAN_POINT ( 'NONE',  ( -79.64356964374999848, -34.97812499938548569, 99.99999999999998579 ) ) ;
#14142=CARTESIAN_POINT ( 'NONE',  ( -85.15643035625001289, -32.84062499938548285, 99.99999999999998579 ) ) ;
#14154=CARTESIAN_POINT ( 'NONE',  ( -82.39999999999999147, -31.85624999877097352, 96.53589838486223584 ) ) ;
#14155=CARTESIAN_POINT ( 'NONE',  ( -79.39999999999999147, -33.73124999877096997, 98.26794919243110371 ) ) ;
#14167=CARTESIAN_POINT ( 'NONE',  ( -79.39999999999999147, -35.15624999877096712, 101.7320508075688537 ) ) ;
#14169=DIRECTION ( 'NONE',  ( 0.000000000000000000, -0.000000000000000000, -1.000000000000000000 ) ) ;
#14170=EDGE_LOOP ( 'NONE', ( #1846, #3114, #6108, #13556 ) ) ;
#14171=CARTESIAN_POINT ( 'NONE',  ( -85.15643035625001289, -30.14062499938548711, 99.99999999999998579 ) ) ;
#14173=EDGE_LOOP ( 'NONE', ( #5161, #6779, #16803, #9904 ) ) ;
#14178=CARTESIAN_POINT ( 'NONE',  ( -80.90000000000000568, -30.60000000000000142, 97.40192378864668399 ) ) ;
#14182=FACE_OUTER_BOUND ( 'NONE', #632, .T. ) ;
#14189=CARTESIAN_POINT ( 'NONE',  ( -82.40000000000001990, -33.88124999877096855, 103.0000000000000000 ) ) ;
#14191=CARTESIAN_POINT ( 'NONE',  ( -79.64356964374999848, -33.62812499938548427, 99.99999999999998579 ) ) ;
#14198=VECTOR ( 'NONE', #15302, 1000.000000000000000 ) ;
#14200=CARTESIAN_POINT ( 'NONE',  ( -82.39999999999999147, -32.84062499938548996, 103.1828516163667899 ) ) ;
#14209=CARTESIAN_POINT ( 'NONE',  ( -79.39999999999999147, -34.27499999999999858, 99.99999999999998579 ) ) ;
#14235=CARTESIAN_POINT ( 'NONE',  ( -79.64356964375001269, -33.02812499938548285, 98.40857419181659793 ) ) ;
#14246=CARTESIAN_POINT ( 'NONE',  ( -80.90000000000000568, -32.04374999877096997, 102.5980762113533018 ) ) ;
#14247=CARTESIAN_POINT ( 'NONE',  ( -83.90000000000000568, -35.26874999877097139, 102.5980762113533018 ) ) ;
#14260=CARTESIAN_POINT ( 'NONE',  ( -81.71550957129744575, -35.02336225948853610, 96.93108911813138207 ) ) ;
#14261=CARTESIAN_POINT ( 'NONE',  ( -79.64356964374998427, -30.77812499938548285, 98.40857419181659793 ) ) ;
#14265=CARTESIAN_POINT ( 'NONE',  ( -80.90000000000000568, -33.84374999877096712, 102.5980762113533018 ) ) ;
#14269=CARTESIAN_POINT ( 'NONE',  ( -82.40000000000000568, -30.00000000000000355, 99.99999999999998579 ) ) ;
#14273=CARTESIAN_POINT ( 'NONE',  ( -83.90000000000000568, -34.12106250001229313, 97.40192378864668399 ) ) ;
#14288=CARTESIAN_POINT ( 'NONE',  ( -85.15643035624999868, -34.71562499938548285, 101.5914258081833879 ) ) ;
#14291=CARTESIAN_POINT ( 'NONE',  ( -81.94448577231695197, -35.00123065787786913, 97.01484129690837221 ) ) ;
#14293=EDGE_CURVE ( 'NONE', #2327, #11976, #18602, .T. ) ;
#14294=CARTESIAN_POINT ( 'NONE',  ( -84.51155491706698797, -35.14114833091483803, 98.22820877610629964 ) ) ;
#14299=CARTESIAN_POINT ( 'NONE',  ( -82.39999999999999147, -34.41562499938548569, 96.81714838363319586 ) ) ;
#14309=CARTESIAN_POINT ( 'NONE',  ( -80.90000000000000568, -33.00000000000000000, 102.5980762113533018 ) ) ;
#14317=CARTESIAN_POINT ( 'NONE',  ( -80.90000000000000568, -30.74606250001229313, 102.5980762113533018 ) ) ;
#14321=CARTESIAN_POINT ( 'NONE',  ( -83.90000000000000568, -33.52499999999999858, 102.5980762113533018 ) ) ;
#14324=EDGE_CURVE ( 'NONE', #16645, #4020, #11230, .T. ) ;
#14332=CARTESIAN_POINT ( 'NONE',  ( -82.39999999999999147, -34.75312499938549138, 96.81714838363319586 ) ) ;
#14342=CARTESIAN_POINT ( 'NONE',  ( -79.39999999999999147, -34.70624999877097139, 101.7320508075688537 ) ) ;
#14343=CARTESIAN_POINT ( 'NONE',  ( -83.77821517812500929, -30.77812499938548640, 97.61286128772489690 ) ) ;
#14347=DIRECTION ( 'NONE',  ( -0.000000000000000000, -1.000000000000000000, -0.000000000000000000 ) ) ;
#14356=CARTESIAN_POINT ( 'NONE',  ( -83.77821517812500929, -31.11562499938548498, 97.61286128772489690 ) ) ;
#14363=( LENGTH_UNIT ( ) NAMED_UNIT ( * ) SI_UNIT ( .MILLI., .METRE. ) );
#14367=CARTESIAN_POINT ( 'NONE',  ( -79.39999999999999147, -32.06250000000000000, 101.7320508075688537 ) ) ;
#14377=CYLINDRICAL_SURFACE ( 'NONE', #14574, 3.000000000000002665 ) ;
#14378=CARTESIAN_POINT ( 'NONE',  ( -82.40000000000000568, -30.00000000000000355, 96.99999999999998579 ) ) ;
#14380=CARTESIAN_POINT ( 'NONE',  ( -83.77821517812500929, -33.02812499938548285, 97.61286128772489690 ) ) ;
#14384=CARTESIAN_POINT ( 'NONE',  ( -85.15643035625001289, -34.19062499938548427, 99.99999999999998579 ) ) ;
#14389=CARTESIAN_POINT ( 'NONE',  ( -83.77821517812500929, -33.47812499938548569, 97.61286128772489690 ) ) ;
#14398=DIRECTION ( 'NONE',  ( 0.000000000000000000, 0.000000000000000000, -1.000000000000000000 ) ) ;
#14400=CARTESIAN_POINT ( 'NONE',  ( -79.39999999999999147, -33.41250000000000142, 101.7320508075688537 ) ) ;
#14407=LINE ( 'NONE', #12951, #13904 ) ;
#14409=LINE ( 'NONE', #1236, #5175 ) ;
#14425=CARTESIAN_POINT ( 'NONE',  ( -79.64356964375001269, -34.82812499938548711, 98.40857419181659793 ) ) ;
#14435=CARTESIAN_POINT ( 'NONE',  ( -83.90000000000000568, -35.26874999877097139, 102.5980762113533018 ) ) ;
#14436=CARTESIAN_POINT ( 'NONE',  ( -82.39999999999999147, -31.94062499938548427, 103.1828516163667899 ) ) ;
#14448=CARTESIAN_POINT ( 'NONE',  ( -79.64356964374998427, -30.85312499938548569, 101.5914258081833879 ) ) ;
#14451=CARTESIAN_POINT ( 'NONE',  ( -81.59615242270662350, -31.87634618820330701, 97.00000000000000000 ) ) ;
#14453=VERTEX_POINT ( 'NONE', #15049 ) ;
#14457=CARTESIAN_POINT ( 'NONE',  ( -79.39999999999999147, -31.53750000000000497, 98.26794919243110371 ) ) ;
#14471=CARTESIAN_POINT ( 'NONE',  ( -85.15643035624999868, -33.44062499938548427, 98.40857419181659793 ) ) ;
#14476=CARTESIAN_POINT ( 'NONE',  ( -81.02178482187500208, -33.59062499938548285, 102.3871387122750889 ) ) ;
#14482=CARTESIAN_POINT ( 'NONE',  ( -82.39999999999999147, -33.74062499938548854, 103.1828516163667899 ) ) ;
#14494=CARTESIAN_POINT ( 'NONE',  ( -82.39999999999999147, -32.58750000000000568, 103.4641016151377499 ) ) ;
#14499=MECHANICAL_DESIGN_GEOMETRIC_PRESENTATION_REPRESENTATION('',(#806),#13571);
#14503=CARTESIAN_POINT ( 'NONE',  ( -79.39999999999999147, -34.72500000000000142, 99.99999999999998579 ) ) ;
#14505=CARTESIAN_POINT ( 'NONE',  ( -82.39999999999999147, -30.25312499938548783, 96.81714838363319586 ) ) ;
#14520=DIRECTION ( 'NONE',  ( 0.000000000000000000, 0.000000000000000000, -1.000000000000000000 ) ) ;
#14524=DIRECTION ( 'NONE',  ( 0.000000000000000000, 0.000000000000000000, -1.000000000000000000 ) ) ;
#14532=CARTESIAN_POINT ( 'NONE',  ( -79.39999999999999147, -30.58518749875867826, 98.26794919243110371 ) ) ;
#14533=CARTESIAN_POINT ( 'NONE',  ( -79.64356964375001269, -31.41562499938548569, 101.5914258081833879 ) ) ;
#14546=CARTESIAN_POINT ( 'NONE',  ( -82.39999999999999147, -34.83749999999999858, 103.0000000000000000 ) ) ;
#14553=CARTESIAN_POINT ( 'NONE',  ( -83.90000000000000568, -30.97500000000000142, 97.40192378864668399 ) ) ;
#14560=AXIS2_PLACEMENT_3D ( 'NONE', #10706, #9234, #1816 ) ;
#14567=CARTESIAN_POINT ( 'NONE',  ( -82.39999999999999147, -30.25312499938548783, 96.81714838363319586 ) ) ;
#14571=CARTESIAN_POINT ( 'NONE',  ( -83.77821517812500929, -32.91562499938547859, 97.61286128772489690 ) ) ;
#14574=AXIS2_PLACEMENT_3D ( 'NONE', #12920, #4221, #5511 ) ;
#14594=CARTESIAN_POINT ( 'NONE',  ( -80.90000000000000568, -33.89999999999999858, 102.5980762113533018 ) ) ;
#14600=VECTOR ( 'NONE', #5502, 1000.000000000000000 ) ;
#14604=CARTESIAN_POINT ( 'NONE',  ( -83.90000000000000568, -30.52106250001229526, 97.40192378864668399 ) ) ;
#14607=CARTESIAN_POINT ( 'NONE',  ( -82.39999999999999147, -31.37812499938548427, 103.1828516163667899 ) ) ;
#14608=CARTESIAN_POINT ( 'NONE',  ( -85.40000000000000568, -32.64374999877097139, 99.99999999999998579 ) ) ;
#14625=CARTESIAN_POINT ( 'NONE',  ( -85.40000000000000568, -32.19374999877096855, 99.99999999999998579 ) ) ;
#14630=CARTESIAN_POINT ( 'NONE',  ( -85.40000000000000568, -33.99374999877097281, 99.99999999999998579 ) ) ;
#14631=CARTESIAN_POINT ( 'NONE',  ( -83.77821517812500929, -31.07812499938548711, 102.3871387122750889 ) ) ;
#14634=( BOUNDED_CURVE ( )  B_SPLINE_CURVE ( 2, ( #12905, #5197, #2454, #2255, #18775, #11144, #14265, #619, #714 ),
 .UNSPECIFIED., .F., .F. ) 
 B_SPLINE_CURVE_WITH_KNOTS ( ( 3, 2, 2, 2, 3 ),
 ( 0.6041666666666665186, 0.6111111111111111605, 0.6250000000000000000, 0.6388888888888888395, 0.6458333333333333703 ),
 .UNSPECIFIED. ) 
 CURVE ( )  GEOMETRIC_REPRESENTATION_ITEM ( )  RATIONAL_B_SPLINE_CURVE ( ( 0.9330127018922194093, 0.9330127018922177440, 1.000000000000000000, 0.8660254037844387076, 1.000000000000000000, 0.8660254037844387076, 1.000000000000000000, 0.9330127018922187432, 0.9330127018922192983 ) ) 
 REPRESENTATION_ITEM ( '' )  );
#14643=CARTESIAN_POINT ( 'NONE',  ( -85.15643035625001289, -31.07812499938548356, 98.40857419181659793 ) ) ;
#14647=CARTESIAN_POINT ( 'NONE',  ( -82.40000000000000568, -50.00000000000000000, 107.5000000000000142 ) ) ;
#14655=CARTESIAN_POINT ( 'NONE',  ( -82.39999999999999147, -31.46250000000000568, 96.53589838486223584 ) ) ;
#14664=DIRECTION ( 'NONE',  ( 0.000000000000000000, 0.000000000000000000, -1.000000000000000000 ) ) ;
#14666=CARTESIAN_POINT ( 'NONE',  ( -79.39999999999999147, -33.31874999877096855, 99.99999999999998579 ) ) ;
#14668=CARTESIAN_POINT ( 'NONE',  ( -85.15643035625001289, -35.20312499938548711, 99.99999999999998579 ) ) ;
#14674=CARTESIAN_POINT ( 'NONE',  ( -81.02178482187500208, -34.94062499938548427, 102.3871387122750889 ) ) ;
#14681=CARTESIAN_POINT ( 'NONE',  ( -81.59615242270662350, -30.58259618943234059, 96.99999999999998579 ) ) ;
#14687=ORIENTED_EDGE ( 'NONE', *, *, #7074, .T. ) ;
#14689=CARTESIAN_POINT ( 'NONE',  ( -83.90000000000000568, -34.96874999877096712, 97.40192378864668399 ) ) ;
#14696=CARTESIAN_POINT ( 'NONE',  ( -79.39999999999999147, -32.50856250001229597, 101.7320508075688537 ) ) ;
#14700=CARTESIAN_POINT ( 'NONE',  ( -85.15643035624999868, -31.90312499938548285, 101.5914258081833879 ) ) ;
#14725=CARTESIAN_POINT ( 'NONE',  ( -80.90000000000000568, -34.29374999877096997, 102.5980762113533018 ) ) ;
#14726=CARTESIAN_POINT ( 'NONE',  ( -85.15643035624999868, -32.91562499938549280, 101.5914258081833879 ) ) ;
#14731=EDGE_CURVE ( 'NONE', #18235, #2812, #15921, .T. ) ;
#14734=EDGE_CURVE ( 'NONE', #16323, #13062, #9864, .T. ) ;
#14740=CARTESIAN_POINT ( 'NONE',  ( -79.64356964374998427, -32.65312499938548285, 101.5914258081833879 ) ) ;
#14745=CARTESIAN_POINT ( 'NONE',  ( -82.39999999999999147, -34.33124999877097139, 103.0000000000000000 ) ) ;
#14753=CARTESIAN_POINT ( 'NONE',  ( -80.90000000000000568, -33.00000000000000000, 102.5980762113533018 ) ) ;
#14755=CARTESIAN_POINT ( 'NONE',  ( -82.39999999999999147, -30.95624999877097139, 96.53589838486223584 ) ) ;
#14756=CARTESIAN_POINT ( 'NONE',  ( -82.40000000000000568, -30.33749999999999858, 102.9999999999999858 ) ) ;
#14767=CARTESIAN_POINT ( 'NONE',  ( -81.02178482187500208, -30.89062499938548711, 102.3871387122750889 ) ) ;
#14768=PLANE ( 'NONE',  #5068 ) ;
#14774=CARTESIAN_POINT ( 'NONE',  ( -85.40000000000000568, -32.28750000000000142, 98.26794919243111792 ) ) ;
#14779=CARTESIAN_POINT ( 'NONE',  ( -85.40000000000000568, -32.70000000000000284, 99.99999999999998579 ) ) ;
#14786=CARTESIAN_POINT ( 'NONE',  ( -79.39999999999999147, -31.51874999877096784, 99.99999999999998579 ) ) ;
#14797=CARTESIAN_POINT ( 'NONE',  ( -82.39999999999999147, -31.45856250001229881, 96.53589838486223584 ) ) ;
#14800=CARTESIAN_POINT ( 'NONE',  ( -81.02178482187500208, -31.64062499938548356, 97.61286128772489690 ) ) ;
#14807=EDGE_LOOP ( 'NONE', ( #16312, #17826, #10463 ) ) ;
#14815=( BOUNDED_CURVE ( )  B_SPLINE_CURVE ( 2, ( #6353, #6548, #10934, #16804, #12306, #16610, #3217, #16516, #12493 ),
 .UNSPECIFIED., .F., .F. ) 
 B_SPLINE_CURVE_WITH_KNOTS ( ( 3, 2, 2, 2, 3 ),
 ( 0.1458333333333334814, 0.1527777777777777901, 0.1666666666666666574, 0.1805555555555555525, 0.1875000000000000278 ),
 .UNSPECIFIED. ) 
 CURVE ( )  GEOMETRIC_REPRESENTATION_ITEM ( )  RATIONAL_B_SPLINE_CURVE ( ( 0.9330127018922194093, 0.9330127018922207416, 1.000000000000000000, 0.8660254037844387076, 1.000000000000000000, 0.8660254037844387076, 1.000000000000000000, 0.9330127018922190762, 0.9330127018922194093 ) ) 
 REPRESENTATION_ITEM ( '' )  );
#14822=CARTESIAN_POINT ( 'NONE',  ( -83.90000000000000568, -31.37268749875867613, 97.40192378864668399 ) ) ;
#14824=CARTESIAN_POINT ( 'NONE',  ( -82.39999999999999147, -33.29062499938549280, 103.1828516163667899 ) ) ;
#14832=EDGE_CURVE ( 'NONE', #9677, #11976, #2605, .T. ) ;
#14837=CARTESIAN_POINT ( 'NONE',  ( -85.15643035625001289, -33.70312499938548711, 101.5914258081833879 ) ) ;
#14849=CARTESIAN_POINT ( 'NONE',  ( -85.40000000000000568, -34.95000000000000284, 99.99999999999998579 ) ) ;
#14851=CARTESIAN_POINT ( 'NONE',  ( -85.40000000000000568, -30.43124999877096926, 98.26794919243111792 ) ) ;
#14855=FACE_OUTER_BOUND ( 'NONE', #3613, .T. ) ;
#14864=CARTESIAN_POINT ( 'NONE',  ( -83.77821517812500929, -31.86562499938548498, 102.3871387122750889 ) ) ;
#14865=CARTESIAN_POINT ( 'NONE',  ( -85.40000000000000568, -34.05000000000000426, 99.99999999999998579 ) ) ;
#14867=DIRECTION ( 'NONE',  ( -0.000000000000000000, -1.000000000000000000, -0.000000000000000000 ) ) ;
#14871=CARTESIAN_POINT ( 'NONE',  ( -83.90000000000000568, -31.72500000000000142, 102.5980762113533018 ) ) ;
#14886=VERTEX_POINT ( 'NONE', #4579 ) ;
#14889=CARTESIAN_POINT ( 'NONE',  ( -84.01447415327271528, -35.02670941564510088, 97.25687757881057394 ) ) ;
#14891=VERTEX_POINT ( 'NONE', #11811 ) ;
#14896=CARTESIAN_POINT ( 'NONE',  ( -85.40000000000000568, -32.73356250001228318, 98.26794919243111792 ) ) ;
#14902=CARTESIAN_POINT ( 'NONE',  ( -79.64356964374999848, -31.71562499938548285, 99.99999999999998579 ) ) ;
#14908=DIRECTION ( 'NONE',  ( -0.000000000000000000, -1.000000000000000000, -0.000000000000000000 ) ) ;
#14910=EDGE_LOOP ( 'NONE', ( #2090, #8695, #14943, #5127 ) ) ;
#14915=CARTESIAN_POINT ( 'NONE',  ( -83.90000000000000568, -33.07500000000000284, 102.5980762113533018 ) ) ;
#14928=CARTESIAN_POINT ( 'NONE',  ( -82.39999999999999147, -32.76018749875868252, 96.53589838486223584 ) ) ;
#14930=CARTESIAN_POINT ( 'NONE',  ( -82.39999999999999147, -34.41562499938547859, 96.81714838363319586 ) ) ;
#14932=CARTESIAN_POINT ( 'NONE',  ( -81.59615242270662350, -31.66740381056766651, 103.0000000000000000 ) ) ;
#14942=CARTESIAN_POINT ( 'NONE',  ( -82.39999999999999147, -34.52812499938548285, 103.1828516163667899 ) ) ;
#14943=ORIENTED_EDGE ( 'NONE', *, *, #9865, .F. ) ;
#14950=CARTESIAN_POINT ( 'NONE',  ( -82.40000000000001990, -33.65624999877097423, 97.00000000000000000 ) ) ;
#14952=CARTESIAN_POINT ( 'NONE',  ( -85.40000000000000568, -34.53750000000000142, 98.26794919243111792 ) ) ;
#14953=CARTESIAN_POINT ( 'NONE',  ( -80.90000000000000568, -32.34374999877096712, 97.40192378864668399 ) ) ;
#14954=DIRECTION ( 'NONE',  ( 0.000000000000000000, -1.000000000000000000, 0.000000000000000000 ) ) ;
#14967=CARTESIAN_POINT ( 'NONE',  ( -82.39999999999999147, -35.09062499938548285, 103.1828516163667899 ) ) ;
#14970=ORIENTED_EDGE ( 'NONE', *, *, #7133, .T. ) ;
#14973=CARTESIAN_POINT ( 'NONE',  ( -82.39999999999999147, -30.11250000000000426, 96.53589838486223584 ) ) ;
#14985=CARTESIAN_POINT ( 'NONE',  ( -82.40000000000000568, -31.63124999877096855, 102.9999999999999858 ) ) ;
#14991=EDGE_CURVE ( 'NONE', #11600, #12396, #16502, .T. ) ;
#14993=ORIENTED_EDGE ( 'NONE', *, *, #11010, .T. ) ;
#14998=CARTESIAN_POINT ( 'NONE',  ( -85.40000000000000568, -32.20856250001229171, 101.7320508075688679 ) ) ;
#15002=CARTESIAN_POINT ( 'NONE',  ( -83.77821517812500929, -31.86562499938548498, 102.3871387122750889 ) ) ;
#15015=VERTEX_POINT ( 'NONE', #6433 ) ;
#15023=CARTESIAN_POINT ( 'NONE',  ( -82.39999999999999147, -32.31018749875868679, 96.53589838486223584 ) ) ;
#15024=CARTESIAN_POINT ( 'NONE',  ( -81.02178482187500208, -32.65312499938548996, 97.61286128772489690 ) ) ;
#15035=CARTESIAN_POINT ( 'NONE',  ( -85.15643035625001289, -33.25312499938548427, 101.5914258081833879 ) ) ;
#15037=ORIENTED_EDGE ( 'NONE', *, *, #6848, .T. ) ;
#15039=CARTESIAN_POINT ( 'NONE',  ( -79.39999999999999147, -34.25624999877096855, 101.7320508075688537 ) ) ;
#15042=DIRECTION ( 'NONE',  ( 0.000000000000000000, 0.000000000000000000, -1.000000000000000000 ) ) ;
#15043=CARTESIAN_POINT ( 'NONE',  ( -82.39999999999999147, -31.85624999877096641, 96.99999999999998579 ) ) ;
#15046=CARTESIAN_POINT ( 'NONE',  ( -79.39999999999999147, -30.61874999877096926, 99.99999999999998579 ) ) ;
#15047=CARTESIAN_POINT ( 'NONE',  ( -85.40000000000000568, -32.64374999877097139, 99.99999999999998579 ) ) ;
#15049=CARTESIAN_POINT ( 'NONE',  ( -82.39999999999999147, -31.01249999999999929, 96.99999999999998579 ) ) ;
#15056=VECTOR ( 'NONE', #17525, 1000.000000000000000 ) ;
#15060=CARTESIAN_POINT ( 'NONE',  ( -85.15643035624999868, -33.77812499938548285, 98.40857419181659793 ) ) ;
#15064=ORIENTED_EDGE ( 'NONE', *, *, #6390, .F. ) ;
#15066=CARTESIAN_POINT ( 'NONE',  ( -80.90000000000000568, -31.20000000000000284, 102.5980762113533018 ) ) ;
#15074=ADVANCED_FACE ( 'NONE', ( #767 ), #8086, .T. ) ;
#15083=CARTESIAN_POINT ( 'NONE',  ( -82.40000000000001990, -34.61250000000001137, 97.00000000000000000 ) ) ;
#15090=CARTESIAN_POINT ( 'NONE',  ( -82.39999999999999147, -33.03356250001230165, 103.4641016151377499 ) ) ;
#15094=CARTESIAN_POINT ( 'NONE',  ( -81.02178482187500208, -30.55312499938548854, 102.3871387122750889 ) ) ;
#15115=CARTESIAN_POINT ( 'NONE',  ( -85.40000000000000568, -31.29768749875867684, 99.99999999999998579 ) ) ;
#15116=ORIENTED_EDGE ( 'NONE', *, *, #7661, .F. ) ;
#15117=CARTESIAN_POINT ( 'NONE',  ( -81.02178482187500208, -33.25312499938548427, 102.3871387122750889 ) ) ;
#15126=VERTEX_POINT ( 'NONE', #12385 ) ;
#15138=CYLINDRICAL_SURFACE ( 'NONE', #2649, 3.000000000000002665 ) ;
#15142=CARTESIAN_POINT ( 'NONE',  ( -85.40000000000000568, -33.63750000000000284, 98.26794919243111792 ) ) ;
#15143=CARTESIAN_POINT ( 'NONE',  ( -82.39999999999999147, -31.40624999877097068, 96.53589838486223584 ) ) ;
#15144=DIRECTION ( 'NONE',  ( 0.000000000000000000, 0.000000000000000000, -1.000000000000000000 ) ) ;
#15160=CARTESIAN_POINT ( 'NONE',  ( -80.90000000000000568, -30.30000000000000426, 102.5980762113533018 ) ) ;
#15165=AXIS2_PLACEMENT_3D ( 'NONE', #9543, #765, #16880 ) ;
#15176=CARTESIAN_POINT ( 'NONE',  ( -82.39999999999999147, -32.16562499938549280, 96.81714838363319586 ) ) ;
#15179=ORIENTED_EDGE ( 'NONE', *, *, #8646, .F. ) ;
#15180=CARTESIAN_POINT ( 'NONE',  ( -84.23541345008663939, -34.99840151550829859, 102.3957176879168713 ) ) ;
#15185=CARTESIAN_POINT ( 'NONE',  ( -85.15643035625001289, -31.11562499938548143, 101.5914258081833879 ) ) ;
#15187=CARTESIAN_POINT ( 'NONE',  ( -82.40000000000000568, -33.03750000000000142, 102.9999999999999858 ) ) ;
#15191=DIRECTION ( 'NONE',  ( -0.000000000000000000, -1.000000000000000000, -0.000000000000000000 ) ) ;
#15196=CARTESIAN_POINT ( 'NONE',  ( -83.20384757729337366, -33.18615380933864145, 97.00000000000000000 ) ) ;
#15201=ORIENTED_EDGE ( 'NONE', *, *, #9496, .F. ) ;
#15211=CARTESIAN_POINT ( 'NONE',  ( -85.40000000000000568, -32.19768749875867542, 99.99999999999998579 ) ) ;
#15240=CARTESIAN_POINT ( 'NONE',  ( -79.39999999999999147, -34.27499999999999858, 99.99999999999998579 ) ) ;
#15241=CARTESIAN_POINT ( 'NONE',  ( -83.90000000000000568, -33.67500000000000426, 97.40192378864668399 ) ) ;
#15242=CARTESIAN_POINT ( 'NONE',  ( -83.90000000000000568, -34.36874999877097281, 102.5980762113533018 ) ) ;
#15251=( LENGTH_UNIT ( ) NAMED_UNIT ( * ) SI_UNIT ( .MILLI., .METRE. ) );
#15273=CARTESIAN_POINT ( 'NONE',  ( -83.90000000000000568, -30.97500000000000142, 97.40192378864668399 ) ) ;
#15276=CARTESIAN_POINT ( 'NONE',  ( -85.15643035625001289, -31.15312499938548996, 99.99999999999998579 ) ) ;
#15280=CARTESIAN_POINT ( 'NONE',  ( -85.11710442811005350, -34.99993311519780548, 101.3183887536204537 ) ) ;
#15284=CARTESIAN_POINT ( 'NONE',  ( -79.64356964374998427, -32.24062499938548854, 98.40857419181659793 ) ) ;
#15294=CARTESIAN_POINT ( 'NONE',  ( -85.40000000000000568, -33.13124999877096855, 98.26794919243111792 ) ) ;
#15302=DIRECTION ( 'NONE',  ( -0.000000000000000000, -1.000000000000000000, -0.000000000000000000 ) ) ;
#15306=CARTESIAN_POINT ( 'NONE',  ( -79.39999999999999147, -33.32268749875867542, 99.99999999999998579 ) ) ;
#15330=CARTESIAN_POINT ( 'NONE',  ( -80.90000000000000568, -31.94999999999999929, 97.40192378864668399 ) ) ;
#15331=CARTESIAN_POINT ( 'NONE',  ( -83.90000000000000568, -31.36874999877096926, 97.40192378864668399 ) ) ;
#15332=CARTESIAN_POINT ( 'NONE',  ( -79.39999999999999147, -33.31874999877096855, 99.99999999999998579 ) ) ;
#15342=SURFACE_STYLE_FILL_AREA ( #327 ) ;
#15346=CYLINDRICAL_SURFACE ( 'NONE', #18951, 7.500000000000020428 ) ;
#15353=ORIENTED_EDGE ( 'NONE', *, *, #10956, .T. ) ;
#15373=CARTESIAN_POINT ( 'NONE',  ( -79.64356964375001269, -30.44062499938548783, 98.40857419181659793 ) ) ;
#15377=CARTESIAN_POINT ( 'NONE',  ( -84.93364891667351912, -34.99959809868389016, 98.35626849035328689 ) ) ;
#15380=CARTESIAN_POINT ( 'NONE',  ( -80.90000000000000568, -34.74374999877097281, 102.5980762113533018 ) ) ;
#15384=( BOUNDED_CURVE ( )  B_SPLINE_CURVE ( 2, ( #4560, #3181, #14915, #7676, #17950, #371, #6127, #6322, #10517 ),
 .UNSPECIFIED., .F., .F. ) 
 B_SPLINE_CURVE_WITH_KNOTS ( ( 3, 2, 2, 2, 3 ),
 ( 0.5625000000000000000, 0.5694444444444444198, 0.5833333333333333703, 0.5972222222222222099, 0.6041666666666666297 ),
 .UNSPECIFIED. ) 
 CURVE ( )  GEOMETRIC_REPRESENTATION_ITEM ( )  RATIONAL_B_SPLINE_CURVE ( ( 0.9330127018922194093, 0.9330127018922194093, 1.000000000000000000, 0.8660254037844387076, 1.000000000000000000, 0.8660254037844387076, 1.000000000000000000, 0.9330127018922198534, 0.9330127018922192983 ) ) 
 REPRESENTATION_ITEM ( '' )  );
#15385=CARTESIAN_POINT ( 'NONE',  ( -82.39999999999999147, -31.71562499938548640, 96.81714838363319586 ) ) ;
#15406=CARTESIAN_POINT ( 'NONE',  ( -79.39999999999999147, -34.26018749875867542, 101.7320508075688537 ) ) ;
#15412=DIRECTION ( 'NONE',  ( -0.000000000000000000, -1.000000000000000000, -0.000000000000000000 ) ) ;
#15418=PRODUCT_CONTEXT ( 'NONE', #7067, 'mechanical' ) ;
#15421=CARTESIAN_POINT ( 'NONE',  ( -82.39999999999999147, -32.72812499938548569, 103.1828516163667899 ) ) ;
#15432=CARTESIAN_POINT ( 'NONE',  ( -85.40000000000000568, -32.68124999877097281, 98.26794919243111792 ) ) ;
#15433=CARTESIAN_POINT ( 'NONE',  ( -83.90000000000000568, -34.96874999877096712, 97.40192378864668399 ) ) ;
#15434=CARTESIAN_POINT ( 'NONE',  ( -82.40000000000000568, -50.00000000000000000, 107.5000000000000142 ) ) ;
#15444=PLANE ( 'NONE',  #12705 ) ;
#15461=CARTESIAN_POINT ( 'NONE',  ( -79.39999999999999147, -34.72106250001229455, 99.99999999999998579 ) ) ;
#15469=ORIENTED_EDGE ( 'NONE', *, *, #15736, .F. ) ;
#15474=CARTESIAN_POINT ( 'NONE',  ( -85.15643035625001289, -30.25312499938548783, 99.99999999999998579 ) ) ;
#15483=CARTESIAN_POINT ( 'NONE',  ( -85.15643035625001289, -30.25312499938548783, 99.99999999999998579 ) ) ;
#15500=PRODUCT_DEFINITION_FORMATION_WITH_SPECIFIED_SOURCE ( 'ANY', '', #12465, .NOT_KNOWN. ) ;
#15502=CARTESIAN_POINT ( 'NONE',  ( -83.20384757729335945, -30.09240381056766722, 96.99999999999998579 ) ) ;
#15505=CARTESIAN_POINT ( 'NONE',  ( -85.40000000000000568, -34.41018749875868821, 101.7320508075688679 ) ) ;
#15506=CARTESIAN_POINT ( 'NONE',  ( -83.77821517812500929, -34.82812499938548711, 97.61286128772489690 ) ) ;
#15521=CARTESIAN_POINT ( 'NONE',  ( -85.15643035624999868, -32.87812499938549138, 98.40857419181659793 ) ) ;
#15526=CYLINDRICAL_SURFACE ( 'NONE', #2868, 3.000000000000002665 ) ;
#15532=CARTESIAN_POINT ( 'NONE',  ( -79.39999999999999147, -33.82500000000000284, 99.99999999999998579 ) ) ;
#15533=CARTESIAN_POINT ( 'NONE',  ( -79.39999999999999147, -31.06874999877096855, 99.99999999999998579 ) ) ;
#15534=CARTESIAN_POINT ( 'NONE',  ( -82.39999999999999147, -33.65624999877096712, 96.53589838486223584 ) ) ;
#15547=FACE_OUTER_BOUND ( 'NONE', #10859, .T. ) ;
#15559=CARTESIAN_POINT ( 'NONE',  ( -85.40000000000000568, -30.03750000000000497, 98.26794919243111792 ) ) ;
#15568=ORIENTED_EDGE ( 'NONE', *, *, #7133, .F. ) ;
#15573=CARTESIAN_POINT ( 'NONE',  ( -79.64356964375001269, -30.89062499938548711, 98.40857419181659793 ) ) ;
#15584=CARTESIAN_POINT ( 'NONE',  ( -85.15643035625001289, -34.30312499938548854, 99.99999999999998579 ) ) ;
#15585=CARTESIAN_POINT ( 'NONE',  ( -82.39999999999999147, -32.81250000000000000, 97.00000000000000000 ) ) ;
#15605=CARTESIAN_POINT ( 'NONE',  ( -80.90000000000000568, -32.94374999877096855, 102.5980762113533018 ) ) ;
#15607=CARTESIAN_POINT ( 'NONE',  ( -82.39999999999999147, -34.78518749875867400, 103.4641016151377499 ) ) ;
#15620=CARTESIAN_POINT ( 'NONE',  ( -79.64356964375001269, -33.92812499938548854, 98.40857419181659793 ) ) ;
#15629=( BOUNDED_CURVE ( )  B_SPLINE_CURVE ( 2, ( #7901, #11118, #11023, #2037, #6447, #10736, #3502, #17086, #7997 ),
 .UNSPECIFIED., .F., .F. ) 
 B_SPLINE_CURVE_WITH_KNOTS ( ( 3, 2, 2, 2, 3 ),
 ( 0.06250000000000006939, 0.06944444444444444753, 0.08333333333333332871, 0.09722222222222222376, 0.1041666666666666713 ),
 .UNSPECIFIED. ) 
 CURVE ( )  GEOMETRIC_REPRESENTATION_ITEM ( )  RATIONAL_B_SPLINE_CURVE ( ( 0.9330127018922194093, 0.9330127018922200755, 1.000000000000000000, 0.8660254037844387076, 1.000000000000000000, 0.8660254037844387076, 1.000000000000000000, 0.9330127018922192983, 0.9330127018922194093 ) ) 
 REPRESENTATION_ITEM ( '' )  );
#15631=CARTESIAN_POINT ( 'NONE',  ( -80.90000000000000568, -32.10000000000000142, 102.5980762113533018 ) ) ;
#15632=CARTESIAN_POINT ( 'NONE',  ( -85.40000000000000568, -33.09374999877096712, 99.99999999999998579 ) ) ;
#15633=CARTESIAN_POINT ( 'NONE',  ( -79.39999999999999147, -34.25624999877096855, 101.7320508075688537 ) ) ;
#15640=( NAMED_UNIT ( * ) SI_UNIT ( $, .STERADIAN. ) SOLID_ANGLE_UNIT ( ) );
#15646=PLANE ( 'NONE',  #9415 ) ;
#15655=CARTESIAN_POINT ( 'NONE',  ( -83.90000000000000568, -30.52500000000000213, 97.40192378864668399 ) ) ;
#15668=CARTESIAN_POINT ( 'NONE',  ( -82.39999999999999147, -34.86562499938548854, 96.81714838363319586 ) ) ;
#15673=CARTESIAN_POINT ( 'NONE',  ( -82.40000000000000568, -34.55624999877097281, 97.00000000000000000 ) ) ;
#15680=CARTESIAN_POINT ( 'NONE',  ( -83.77821517812500929, -34.67812499938548854, 102.3871387122750889 ) ) ;
#15691=CARTESIAN_POINT ( 'NONE',  ( -83.90000000000000568, -33.07500000000000284, 102.5980762113533018 ) ) ;
#15700=CARTESIAN_POINT ( 'NONE',  ( -85.40000000000000568, -30.03356250001229810, 98.26794919243111792 ) ) ;
#15703=CARTESIAN_POINT ( 'NONE',  ( -82.39999999999999147, -33.66018749875868110, 96.53589838486223584 ) ) ;
#15716=CARTESIAN_POINT ( 'NONE',  ( -83.77821517812500929, -33.36562499938548854, 97.61286128772489690 ) ) ;
#15726=CARTESIAN_POINT ( 'NONE',  ( -79.39999999999999147, -32.86874999877097281, 99.99999999999998579 ) ) ;
#15728=CARTESIAN_POINT ( 'NONE',  ( -82.39999999999999147, -32.39062499938548001, 103.1828516163667899 ) ) ;
#15736=EDGE_CURVE ( 'NONE', #14453, #15126, #12597, .T. ) ;
#15741=CARTESIAN_POINT ( 'NONE',  ( -85.15643035625001289, -30.55312499938548143, 101.5914258081833879 ) ) ;
#15742=DIRECTION ( 'NONE',  ( -0.000000000000000000, -1.000000000000000000, -0.000000000000000000 ) ) ;
#15745=DIRECTION ( 'NONE',  ( -0.000000000000000000, 1.000000000000000000, -0.000000000000000000 ) ) ;
#15751=CARTESIAN_POINT ( 'NONE',  ( -83.90000000000000568, -30.07499999999999929, 97.40192378864668399 ) ) ;
#15755=DIRECTION ( 'NONE',  ( 0.000000000000000000, 0.000000000000000000, -1.000000000000000000 ) ) ;
#15764=CARTESIAN_POINT ( 'NONE',  ( -82.39999999999999147, -34.41562499938547859, 96.81714838363319586 ) ) ;
#15766=VERTEX_POINT ( 'NONE', #8420 ) ;
#15767=CARTESIAN_POINT ( 'NONE',  ( -81.44590651011453986, -35.00138974199450814, 97.15054881843455803 ) ) ;
#15768=CARTESIAN_POINT ( 'NONE',  ( -85.15643035624999868, -32.80312499938548854, 101.5914258081833879 ) ) ;
#15769=CARTESIAN_POINT ( 'NONE',  ( -81.59615242270662350, -34.57634618820329564, 96.99999999999997158 ) ) ;
#15774=CARTESIAN_POINT ( 'NONE',  ( -81.02178482187500208, -33.70312499938548711, 102.3871387122750889 ) ) ;
#15784=CARTESIAN_POINT ( 'NONE',  ( -85.40000000000000568, -32.70000000000000284, 99.99999999999998579 ) ) ;
#15795=CARTESIAN_POINT ( 'NONE',  ( -85.40000000000000568, -29.97441297385334025, 100.9999487804559664 ) ) ;
#15821=CARTESIAN_POINT ( 'NONE',  ( -82.40000000000000568, -34.61250000000001137, 97.00000000000000000 ) ) ;
#15822=CARTESIAN_POINT ( 'NONE',  ( -79.39999999999999147, -34.63124999877096855, 98.26794919243110371 ) ) ;
#15824=CARTESIAN_POINT ( 'NONE',  ( -79.64356964374999848, -30.47812499938548569, 99.99999999999998579 ) ) ;
#15836=CARTESIAN_POINT ( 'NONE',  ( -82.65380294351676582, -34.99990492518305274, 97.01075526832239859 ) ) ;
#15837=CARTESIAN_POINT ( 'NONE',  ( -83.77821517812500929, -31.56562499938548427, 97.61286128772489690 ) ) ;
#15850=CARTESIAN_POINT ( 'NONE',  ( -80.90000000000000568, -34.34606250001230165, 102.5980762113533018 ) ) ;
#15864=CARTESIAN_POINT ( 'NONE',  ( -85.15643035624999868, -34.26562499938548711, 101.5914258081833879 ) ) ;
#15867=LINE ( 'NONE', #14647, #4763 ) ;
#15869=CARTESIAN_POINT ( 'NONE',  ( -79.64356964374999848, -33.96562499938548285, 99.99999999999998579 ) ) ;
#15870=LINE ( 'NONE', #19087, #15056 ) ;
#15872=CARTESIAN_POINT ( 'NONE',  ( -85.40000000000000568, -32.66250000000000142, 101.7320508075688821 ) ) ;
#15875=CARTESIAN_POINT ( 'NONE',  ( -85.15643035625001289, -34.75312499938548427, 99.99999999999998579 ) ) ;
#15885=CARTESIAN_POINT ( 'NONE',  ( -79.39999999999999147, -32.51250000000000284, 101.7320508075688537 ) ) ;
#15890=CARTESIAN_POINT ( 'NONE',  ( -85.40000000000000568, -30.85856250001229029, 101.7320508075688679 ) ) ;
#15916=CARTESIAN_POINT ( 'NONE',  ( -79.39999999999999147, -35.15624999877096712, 101.7320508075688537 ) ) ;
#15917=CARTESIAN_POINT ( 'NONE',  ( -79.64356964375001269, -31.86562499938548143, 101.5914258081833879 ) ) ;
#15921=LINE ( 'NONE', #17676, #276 ) ;
#15935=( BOUNDED_CURVE ( )  B_SPLINE_CURVE ( 2, ( #6817, #12468, #12763, #15502, #3964 ),
 .UNSPECIFIED., .F., .F. ) 
 B_SPLINE_CURVE_WITH_KNOTS ( ( 3, 2, 3 ),
 ( 0.000000000000000000, 0.01388888888888888812, 0.02083333333333332871 ),
 .UNSPECIFIED. ) 
 CURVE ( )  GEOMETRIC_REPRESENTATION_ITEM ( )  RATIONAL_B_SPLINE_CURVE ( ( 1.000000000000000000, 0.8660254037844387076, 1.000000000000000000, 0.9330127018922194093, 0.9330127018922191873 ) ) 
 REPRESENTATION_ITEM ( '' )  );
#15941=CARTESIAN_POINT ( 'NONE',  ( -80.90000000000000568, -31.94999999999999929, 97.40192378864668399 ) ) ;
#15954=CARTESIAN_POINT ( 'NONE',  ( -85.15643035624999868, -33.36562499938548854, 101.5914258081833879 ) ) ;
#15957=CARTESIAN_POINT ( 'NONE',  ( -83.77821517812500929, -33.66562499938548569, 102.3871387122750889 ) ) ;
#15964=CARTESIAN_POINT ( 'NONE',  ( -79.64356964374998427, -33.21562499938548996, 101.5914258081833879 ) ) ;
#15967=( BOUNDED_CURVE ( )  B_SPLINE_CURVE ( 2, ( #10307, #16265, #9028, #6005, #11671, #2970, #14689, #1612, #16173 ),
 .UNSPECIFIED., .F., .F. ) 
 B_SPLINE_CURVE_WITH_KNOTS ( ( 3, 2, 2, 2, 3 ),
 ( 0.8125000000000001110, 0.8194444444444444198, 0.8333333333333333703, 0.8472222222222222099, 0.8530683953269213582 ),
 .UNSPECIFIED. ) 
 CURVE ( )  GEOMETRIC_REPRESENTATION_ITEM ( )  RATIONAL_B_SPLINE_CURVE ( ( 0.9330127018922194093, 0.9330127018922204085, 1.000000000000000000, 0.8660254037844387076, 1.000000000000000000, 0.8660254037844387076, 1.000000000000000000, 0.9436068149601996025, 0.9346881722405915305 ) ) 
 REPRESENTATION_ITEM ( '' )  );
#15978=CARTESIAN_POINT ( 'NONE',  ( -79.39999999999999147, -32.43750000000000000, 98.26794919243110371 ) ) ;
#15982=CARTESIAN_POINT ( 'NONE',  ( -85.40000000000000568, -31.35000000000000142, 99.99999999999998579 ) ) ;
#16005=CARTESIAN_POINT ( 'NONE',  ( -85.40000000000000568, -30.00000000000000355, 99.99999999999998579 ) ) ;
#16012=CARTESIAN_POINT ( 'NONE',  ( -79.39999999999999147, -35.08124999877097139, 98.26794919243110371 ) ) ;
#16013=B_SPLINE_CURVE_WITH_KNOTS ( 'NONE', 1,
 ( #3790, #16005 ),
 .UNSPECIFIED., .F., .F.,
 ( 2, 2 ),
 ( 0.000000000000000000, 1.000000000000000000 ),
 .UNSPECIFIED. ) ;
#16014=CARTESIAN_POINT ( 'NONE',  ( -82.39999999999999147, -31.26562499938549067, 96.81714838363319586 ) ) ;
#16026=CARTESIAN_POINT ( 'NONE',  ( -83.77821517812500929, -30.66562499938548569, 97.61286128772489690 ) ) ;
#16037=CARTESIAN_POINT ( 'NONE',  ( -83.90000000000000568, -31.87500000000000000, 97.40192378864668399 ) ) ;
#16050=CARTESIAN_POINT ( 'NONE',  ( -79.64356964375001269, -32.76562499938548711, 101.5914258081833879 ) ) ;
#16054=CARTESIAN_POINT ( 'NONE',  ( -85.15643035625001289, -33.74062499938548854, 99.99999999999998579 ) ) ;
#16058=CARTESIAN_POINT ( 'NONE',  ( -85.40000000000000568, -32.73750000000000426, 98.26794919243111792 ) ) ;
#16068=ORIENTED_EDGE ( 'NONE', *, *, #6653, .T. ) ;
#16069=FACE_OUTER_BOUND ( 'NONE', #11439, .T. ) ;
#16071=CARTESIAN_POINT ( 'NONE',  ( -79.39999999999999147, -33.78750000000000142, 98.26794919243110371 ) ) ;
#16074=ORIENTED_EDGE ( 'NONE', *, *, #11875, .F. ) ;
#16110=CARTESIAN_POINT ( 'NONE',  ( -83.90000000000000568, -34.96874999877096712, 97.40192378864668399 ) ) ;
#16111=CARTESIAN_POINT ( 'NONE',  ( -82.39999999999999147, -30.36562499938549209, 96.81714838363319586 ) ) ;
#16124=CARTESIAN_POINT ( 'NONE',  ( -79.64356964374999848, -30.36562499938548498, 99.99999999999998579 ) ) ;
#16134=CARTESIAN_POINT ( 'NONE',  ( -85.40000000000000568, -32.73750000000000426, 98.26794919243111792 ) ) ;
#16138=CARTESIAN_POINT ( 'NONE',  ( -84.69814109749898989, -35.13162207320847585, 98.07164642868930571 ) ) ;
#16140=( BOUNDED_CURVE ( )  B_SPLINE_CURVE ( 2, ( #502, #1857, #7815, #13963, #6455, #12408, #17579, #11610, #2334 ),
 .UNSPECIFIED., .F., .F. ) 
 B_SPLINE_CURVE_WITH_KNOTS ( ( 3, 2, 2, 2, 3 ),
 ( 0.02083333333333331136, 0.02777777777777777624, 0.04166666666666666435, 0.05555555555555555247, 0.06250000000000006939 ),
 .UNSPECIFIED. ) 
 CURVE ( )  GEOMETRIC_REPRESENTATION_ITEM ( )  RATIONAL_B_SPLINE_CURVE ( ( 0.9330127018922194093, 0.9330127018922191873, 1.000000000000000000, 0.8660254037844387076, 1.000000000000000000, 0.8660254037844387076, 1.000000000000000000, 0.9330127018922187432, 0.9330127018922194093 ) ) 
 REPRESENTATION_ITEM ( '' )  );
#16144=CARTESIAN_POINT ( 'NONE',  ( -80.90000000000000568, -33.24374999877097281, 97.40192378864668399 ) ) ;
#16146=CARTESIAN_POINT ( 'NONE',  ( -85.15643035624999868, -31.97812499938548925, 98.40857419181659793 ) ) ;
#16153=CARTESIAN_POINT ( 'NONE',  ( -81.02178482187500208, -32.99062499938548854, 97.61286128772489690 ) ) ;
#16173=CARTESIAN_POINT ( 'NONE',  ( -82.65380294351676582, -34.99990492518305274, 97.01075526832239859 ) ) ;
#16182=CARTESIAN_POINT ( 'NONE',  ( -79.39999999999999147, -33.40856250001229455, 101.7320508075688537 ) ) ;
#16187=CARTESIAN_POINT ( 'NONE',  ( -79.64356964375001269, -32.20312499938548001, 101.5914258081833879 ) ) ;
#16212=CARTESIAN_POINT ( 'NONE',  ( -82.39999999999999147, -35.00624999877097565, 96.53589838486223584 ) ) ;
#16213=CARTESIAN_POINT ( 'NONE',  ( -81.02178482187500208, -34.00312499938548427, 97.61286128772489690 ) ) ;
#16225=CARTESIAN_POINT ( 'NONE',  ( -85.15643035625001289, -34.15312499938548285, 101.5914258081833879 ) ) ;
#16226=ORIENTED_EDGE ( 'NONE', *, *, #6504, .F. ) ;
#16227=ORIENTED_EDGE ( 'NONE', *, *, #14293, .F. ) ;
#16236=CARTESIAN_POINT ( 'NONE',  ( -83.90000000000000568, -31.42500000000000071, 97.40192378864668399 ) ) ;
#16246=CARTESIAN_POINT ( 'NONE',  ( -79.64356964375001269, -30.85312499938548569, 101.5914258081833879 ) ) ;
#16252=CARTESIAN_POINT ( 'NONE',  ( -79.39999999999999147, -31.57499999999999929, 99.99999999999998579 ) ) ;
#16257=( BOUNDED_CURVE ( )  B_SPLINE_CURVE ( 2, ( #18469, #1952, #697, #18564, #11032, #16996, #3607, #9568, #7910 ),
 .UNSPECIFIED., .F., .F. ) 
 B_SPLINE_CURVE_WITH_KNOTS ( ( 3, 2, 2, 2, 3 ),
 ( 0.3958333333333334259, 0.4027777777777777901, 0.4166666666666666852, 0.4305555555555555802, 0.4375000000000000555 ),
 .UNSPECIFIED. ) 
 CURVE ( )  GEOMETRIC_REPRESENTATION_ITEM ( )  RATIONAL_B_SPLINE_CURVE ( ( 0.9330127018922192983, 0.9330127018922200755, 1.000000000000000000, 0.8660254037844387076, 1.000000000000000000, 0.8660254037844387076, 1.000000000000000000, 0.9330127018922187432, 0.9330127018922192983 ) ) 
 REPRESENTATION_ITEM ( '' )  );
#16263=ORIENTED_EDGE ( 'NONE', *, *, #6848, .F. ) ;
#16265=CARTESIAN_POINT ( 'NONE',  ( -83.20384757729337366, -34.80134618820331127, 103.0000000000000000 ) ) ;
#16272=CARTESIAN_POINT ( 'NONE',  ( -82.40000000000000568, -30.73124999877097352, 103.0000000000000000 ) ) ;
#16273=CARTESIAN_POINT ( 'NONE',  ( -85.40000000000000568, -31.79606250001229384, 99.99999999999998579 ) ) ;
#16278=CARTESIAN_POINT ( 'NONE',  ( -83.77821517812500929, -32.31562499938548427, 102.3871387122750889 ) ) ;
#16283=LINE ( 'NONE', #4658, #16933 ) ;
#16298=CARTESIAN_POINT ( 'NONE',  ( -79.39999999999999147, -30.22500000000000142, 99.99999999999998579 ) ) ;
#16303=CARTESIAN_POINT ( 'NONE',  ( -82.39999999999999147, -32.53518749875867400, 103.4641016151377499 ) ) ;
#16304=CARTESIAN_POINT ( 'NONE',  ( -85.15643035624999868, -34.71562499938548285, 101.5914258081833879 ) ) ;
#16312=ORIENTED_EDGE ( 'NONE', *, *, #5541, .T. ) ;
#16316=CARTESIAN_POINT ( 'NONE',  ( -79.64356964374998427, -33.47812499938547859, 98.40857419181659793 ) ) ;
#16323=VERTEX_POINT ( 'NONE', #18937 ) ;
#16327=CARTESIAN_POINT ( 'NONE',  ( -82.39999999999999147, -31.68750000000000355, 103.4641016151377499 ) ) ;
#16328=CARTESIAN_POINT ( 'NONE',  ( -79.39999999999999147, -32.00624999877096855, 101.7320508075688537 ) ) ;
#16330=ADVANCED_FACE ( 'NONE', ( #13535 ), #19220, .T. ) ;
#16331=CARTESIAN_POINT ( 'NONE',  ( -84.69814181805116959, -35.36146079493983052, 98.07164728741744852 ) ) ;
#16339=CARTESIAN_POINT ( 'NONE',  ( -81.02178482187500208, -31.79062499938548925, 102.3871387122750889 ) ) ;
#16340=CARTESIAN_POINT ( 'NONE',  ( -83.20384757729338787, -33.95759618943233704, 102.9999999999999858 ) ) ;
#16345=CARTESIAN_POINT ( 'NONE',  ( -80.90000000000000568, -31.65000000000000568, 102.5980762113533018 ) ) ;
#16360=DIRECTION ( 'NONE',  ( 0.000000000000000000, 0.000000000000000000, 1.000000000000000000 ) ) ;
#16369=CARTESIAN_POINT ( 'NONE',  ( -83.90000000000000568, -31.27106250001229881, 102.5980762113533018 ) ) ;
#16372=CARTESIAN_POINT ( 'NONE',  ( -82.39999999999999147, -30.92812499938548143, 103.1828516163667899 ) ) ;
#16373=CARTESIAN_POINT ( 'NONE',  ( -79.39999999999999147, -32.96250000000000568, 101.7320508075688537 ) ) ;
#16388=CARTESIAN_POINT ( 'NONE',  ( -81.59615242270662350, -30.13259618943233775, 97.00000000000004263 ) ) ;
#16394=CARTESIAN_POINT ( 'NONE',  ( -85.40000000000000568, -30.88518749875867897, 98.26794919243111792 ) ) ;
#16395=CARTESIAN_POINT ( 'NONE',  ( -83.77821517812500929, -33.32812499938548711, 102.3871387122750889 ) ) ;
#16396=CARTESIAN_POINT ( 'NONE',  ( -79.39999999999999147, -31.61250000000000071, 101.7320508075688537 ) ) ;
#16409=CARTESIAN_POINT ( 'NONE',  ( -79.64356964374998427, -34.37812499938548427, 98.40857419181659793 ) ) ;
#16414=CARTESIAN_POINT ( 'NONE',  ( -85.40000000000000568, -34.91250000000000142, 101.7320508075688821 ) ) ;
#16417=CARTESIAN_POINT ( 'NONE',  ( -83.90000000000000568, -31.81874999877096855, 97.40192378864668399 ) ) ;
#16420=CARTESIAN_POINT ( 'NONE',  ( -79.39999999999999147, -34.27499999999999858, 99.99999999999998579 ) ) ;
#16421=CARTESIAN_POINT ( 'NONE',  ( -85.40000000000000568, -32.19374999877096855, 99.99999999999998579 ) ) ;
#16435=CARTESIAN_POINT ( 'NONE',  ( -81.02178482187500208, -31.34062499938548996, 102.3871387122750889 ) ) ;
#16442=CARTESIAN_POINT ( 'NONE',  ( -83.90000000000000568, -31.27500000000000568, 102.5980762113533018 ) ) ;
#16463=CARTESIAN_POINT ( 'NONE',  ( -83.20384757729335945, -30.35759618943233917, 103.0000000000000000 ) ) ;
#16467=CARTESIAN_POINT ( 'NONE',  ( -79.39999999999999147, -31.57106250001229242, 99.99999999999998579 ) ) ;
#16472=CARTESIAN_POINT ( 'NONE',  ( -81.02178482187500208, -32.54062499938548569, 97.61286128772489690 ) ) ;
#16496=CARTESIAN_POINT ( 'NONE',  ( -79.39999999999999147, -31.56018749875868323, 101.7320508075688537 ) ) ;
#16497=CARTESIAN_POINT ( 'NONE',  ( -79.64356964375001269, -34.04062499938549280, 98.40857419181659793 ) ) ;
#16502=LINE ( 'NONE', #3105, #7396 ) ;
#16509=CARTESIAN_POINT ( 'NONE',  ( -79.64356964374999848, -33.06562499938548427, 99.99999999999998579 ) ) ;
#16510=ORIENTED_EDGE ( 'NONE', *, *, #14734, .T. ) ;
#16516=CARTESIAN_POINT ( 'NONE',  ( -83.20384757729335945, -31.38615380933863008, 96.99999999999997158 ) ) ;
#16520=CARTESIAN_POINT ( 'NONE',  ( -85.40000000000000568, -30.39374999877097139, 99.99999999999998579 ) ) ;
#16521=CARTESIAN_POINT ( 'NONE',  ( -82.39999999999999147, -32.30624999877097281, 96.53589838486223584 ) ) ;
#16522=CARTESIAN_POINT ( 'NONE',  ( -82.40000000000001990, -34.55624999877097281, 97.00000000000000000 ) ) ;
#16533=CARTESIAN_POINT ( 'NONE',  ( -84.69814161231455785, -35.39427329483935836, 98.07164704222795137 ) ) ;
#16534=( BOUNDED_CURVE ( )  B_SPLINE_CURVE ( 2, ( #15836, #14260, #19057, #17398, #2448, #14167, #5586, #8403, #991, #11533, #12803, #12899, #17495 ),
 .UNSPECIFIED., .F., .F. ) 
 B_SPLINE_CURVE_WITH_KNOTS ( ( 3, 2, 2, 2, 2, 2, 3 ),
 ( 0.8530683953269213582, 0.8611111111111111605, 0.8750000000000000000, 0.8888888888888888395, 0.9027777777777777901, 0.9166666666666666297, 0.9258785004222062076 ),
 .UNSPECIFIED. ) 
 CURVE ( )  GEOMETRIC_REPRESENTATION_ITEM ( )  RATIONAL_B_SPLINE_CURVE ( ( 0.9346881722405915305, 0.9224185888242391052, 1.000000000000000000, 0.8660254037844387076, 1.000000000000000000, 0.8660254037844387076, 1.000000000000000000, 0.8660254037844387076, 1.000000000000000000, 0.8660254037844387076, 1.000000000000000000, 0.9111410770381633828, 0.9401538762233125901 ) ) 
 REPRESENTATION_ITEM ( '' )  );
#16536=CARTESIAN_POINT ( 'NONE',  ( -81.02178482187500208, -33.44062499938548427, 97.61286128772489690 ) ) ;
#16543=CARTESIAN_POINT ( 'NONE',  ( -80.90000000000000568, -31.05000000000000071, 97.40192378864668399 ) ) ;
#16561=CARTESIAN_POINT ( 'NONE',  ( -85.34657078790640128, -35.00060087132568754, 100.6622129346251597 ) ) ;
#16565=CARTESIAN_POINT ( 'NONE',  ( -83.90000000000000568, -32.17106250001229739, 102.5980762113533018 ) ) ;
#16589=CARTESIAN_POINT ( 'NONE',  ( -85.40000000000000568, -30.84768749875867755, 99.99999999999998579 ) ) ;
#16590=CARTESIAN_POINT ( 'NONE',  ( -79.64356964374999848, -32.72812499938548569, 99.99999999999998579 ) ) ;
#16603=CARTESIAN_POINT ( 'NONE',  ( -81.02178482187500208, -33.89062499938548711, 97.61286128772489690 ) ) ;
#16610=CARTESIAN_POINT ( 'NONE',  ( -85.40000000000000568, -31.33124999877096784, 98.26794919243111792 ) ) ;
#16614=CARTESIAN_POINT ( 'NONE',  ( -79.39999999999999147, -33.33749999999999858, 98.26794919243110371 ) ) ;
#16615=CARTESIAN_POINT ( 'NONE',  ( -85.40000000000000568, -32.68124999877097281, 98.26794919243111792 ) ) ;
#16622=ORIENTED_EDGE ( 'NONE', *, *, #14991, .F. ) ;
#16635=CARTESIAN_POINT ( 'NONE',  ( -83.90000000000000568, -30.37500000000000355, 102.5980762113533018 ) ) ;
#16645=VERTEX_POINT ( 'NONE', #9632 ) ;
#16651=CARTESIAN_POINT ( 'NONE',  ( -82.39999999999999147, -31.94062499938548427, 103.1828516163667899 ) ) ;
#16654=EDGE_CURVE ( 'NONE', #2034, #15766, #10601, .T. ) ;
#16656=CARTESIAN_POINT ( 'NONE',  ( -79.39542567806877571, -34.99994613746206085, 100.0094913129781560 ) ) ;
#16658=CARTESIAN_POINT ( 'NONE',  ( -80.90000000000000568, -32.40000000000000568, 97.40192378864668399 ) ) ;
#16659=CARTESIAN_POINT ( 'NONE',  ( -79.39999999999999147, -33.85856250001229029, 101.7320508075688537 ) ) ;
#16661=CARTESIAN_POINT ( 'NONE',  ( -82.39999999999999147, -30.81562499938548427, 96.81714838363319586 ) ) ;
#16662=CARTESIAN_POINT ( 'NONE',  ( -84.51155386534844638, -35.25364837475780888, 98.22820752270799005 ) ) ;
#16671=FACE_OUTER_BOUND ( 'NONE', #13634, .T. ) ;
#16682=CARTESIAN_POINT ( 'NONE',  ( -85.40000000000000568, -32.23518749875868394, 98.26794919243111792 ) ) ;
#16706=CARTESIAN_POINT ( 'NONE',  ( -79.39999999999999147, -32.02500000000000568, 99.99999999999998579 ) ) ;
#16707=CARTESIAN_POINT ( 'NONE',  ( -85.40000000000000568, -30.88124999877097210, 98.26794919243111792 ) ) ;
#16708=CARTESIAN_POINT ( 'NONE',  ( -79.39999999999999147, -30.58124999877096784, 98.26794919243110371 ) ) ;
#16720=CARTESIAN_POINT ( 'NONE',  ( -82.40000000000000568, -33.43124999877096570, 102.9999999999999858 ) ) ;
#16740=CARTESIAN_POINT ( 'NONE',  ( -83.90000000000000568, -30.82500000000000284, 102.5980762113533018 ) ) ;
#16742=CARTESIAN_POINT ( 'NONE',  ( -81.02178482187500208, -30.40312499938548640, 97.61286128772489690 ) ) ;
#16745=EDGE_LOOP ( 'NONE', ( #13834, #9981 ) ) ;
#16747=CARTESIAN_POINT ( 'NONE',  ( -84.69814161231455785, -35.39427329483935836, 98.07164704222793716 ) ) ;
#16750=CARTESIAN_POINT ( 'NONE',  ( -82.39999999999999147, -32.39062499938548711, 103.1828516163667899 ) ) ;
#16763=CARTESIAN_POINT ( 'NONE',  ( -82.40000000000001990, -33.20624999877097849, 97.00000000000000000 ) ) ;
#16777=CARTESIAN_POINT ( 'NONE',  ( -82.39999999999999147, -33.43518749875868679, 103.4641016151377499 ) ) ;
#16778=AXIS2_PLACEMENT_3D ( 'NONE', #13584, #12131, #14664 ) ;
#16779=VERTEX_POINT ( 'NONE', #2489 ) ;
#16797=VECTOR ( 'NONE', #2586, 1000.000000000000000 ) ;
#16803=ORIENTED_EDGE ( 'NONE', *, *, #7100, .F. ) ;
#16804=CARTESIAN_POINT ( 'NONE',  ( -85.40000000000000568, -31.25624999877096855, 101.7320508075688821 ) ) ;
#16808=CARTESIAN_POINT ( 'NONE',  ( -79.39999999999999147, -32.38124999877096855, 98.26794919243110371 ) ) ;
#16810=CARTESIAN_POINT ( 'NONE',  ( -79.39999999999999147, -33.80624999877097281, 101.7320508075688537 ) ) ;
#16818=( NAMED_UNIT ( * ) PLANE_ANGLE_UNIT ( ) SI_UNIT ( $, .RADIAN. ) );
#16822=CARTESIAN_POINT ( 'NONE',  ( -82.40000000000000568, -30.00000000000000355, 103.0000000000000000 ) ) ;
#16830=EDGE_LOOP ( 'NONE', ( #10987, #5139, #19084, #5796 ) ) ;
#16836=LINE ( 'NONE', #3442, #8362 ) ;
#16845=CARTESIAN_POINT ( 'NONE',  ( -83.20384757729335945, -34.08615380933863293, 96.99999999999998579 ) ) ;
#16847=CARTESIAN_POINT ( 'NONE',  ( -85.15643035624999868, -32.54062499938548569, 98.40857419181659793 ) ) ;
#16855=CARTESIAN_POINT ( 'NONE',  ( -83.77821517812500929, -31.52812499938548996, 102.3871387122750889 ) ) ;
#16871=EDGE_CURVE ( 'NONE', #2550, #3433, #15967, .T. ) ;
#16874=CARTESIAN_POINT ( 'NONE',  ( -80.90000000000000568, -32.79374999877096997, 97.40192378864668399 ) ) ;
#16876=CARTESIAN_POINT ( 'NONE',  ( -79.39999999999999147, -33.81018749875868679, 101.7320508075688537 ) ) ;
#16879=CARTESIAN_POINT ( 'NONE',  ( -83.90000000000000568, -34.36874999877097281, 102.5980762113533018 ) ) ;
#16880=DIRECTION ( 'NONE',  ( 1.000000000000000000, 0.000000000000000000, -0.000000000000000000 ) ) ;
#16882=( BOUNDED_CURVE ( )  B_SPLINE_CURVE ( 2, ( #3416, #14059, #4892, #5086, #15240, #693, #3704, #12209, #7812 ),
 .UNSPECIFIED., .F., .F. ) 
 B_SPLINE_CURVE_WITH_KNOTS ( ( 3, 2, 2, 2, 3 ),
 ( 0.7708333333333333703, 0.7777777777777777901, 0.7916666666666666297, 0.8055555555555555802, 0.8125000000000000000 ),
 .UNSPECIFIED. ) 
 CURVE ( )  GEOMETRIC_REPRESENTATION_ITEM ( )  RATIONAL_B_SPLINE_CURVE ( ( 0.9330127018922192983, 0.9330127018922198534, 1.000000000000000000, 0.8660254037844387076, 1.000000000000000000, 0.8660254037844387076, 1.000000000000000000, 0.9330127018922194093, 0.9330127018922194093 ) ) 
 REPRESENTATION_ITEM ( '' )  );
#16886=EDGE_CURVE ( 'NONE', #2507, #12906, #11765, .T. ) ;
#16887=EDGE_LOOP ( 'NONE', ( #9434, #19130, #13013, #10549 ) ) ;
#16893=CARTESIAN_POINT ( 'NONE',  ( -82.39999999999999147, -33.40312499938548285, 96.81714838363319586 ) ) ;
#16903=DIRECTION ( 'NONE',  ( -0.000000000000000000, -1.000000000000000000, -0.000000000000000000 ) ) ;
#16904=CARTESIAN_POINT ( 'NONE',  ( -80.90000000000000568, -32.94374999877096855, 102.5980762113533018 ) ) ;
#16905=CARTESIAN_POINT ( 'NONE',  ( -83.90000000000000568, -33.01874999877097139, 102.5980762113533018 ) ) ;
#16913=ORIENTED_EDGE ( 'NONE', *, *, #27, .F. ) ;
#16933=VECTOR ( 'NONE', #15191, 1000.000000000000000 ) ;
#16939=CARTESIAN_POINT ( 'NONE',  ( -85.15643035625001289, -31.60312499938548569, 99.99999999999998579 ) ) ;
#16945=CARTESIAN_POINT ( 'NONE',  ( -81.59615242270662350, -34.76115380933863719, 103.0000000000000000 ) ) ;
#16948=CARTESIAN_POINT ( 'NONE',  ( -85.15643035625001289, -32.05312499938548854, 99.99999999999998579 ) ) ;
#16968=CARTESIAN_POINT ( 'NONE',  ( -79.39999999999999147, -35.16018749875868821, 101.7320508075688537 ) ) ;
#16982=CARTESIAN_POINT ( 'NONE',  ( -85.15643035624999868, -34.15312499938548285, 101.5914258081833879 ) ) ;
#16983=CARTESIAN_POINT ( 'NONE',  ( -79.64356964374999848, -34.86562499938548143, 99.99999999999998579 ) ) ;
#16985=VERTEX_POINT ( 'NONE', #15083 ) ;
#16991=SHAPE_REPRESENTATION ( 'leg', ( #10540 ), #9915 ) ;
#16992=CARTESIAN_POINT ( 'NONE',  ( -82.40000000000000568, -33.71249999999998437, 96.99999999999998579 ) ) ;
#16993=CARTESIAN_POINT ( 'NONE',  ( -83.90000000000000568, -32.71874999877096712, 97.40192378864668399 ) ) ;
#16995=CARTESIAN_POINT ( 'NONE',  ( -79.39999999999999147, -32.86874999877097281, 99.99999999999998579 ) ) ;
#16996=CARTESIAN_POINT ( 'NONE',  ( -85.40000000000000568, -32.28750000000000142, 98.26794919243111792 ) ) ;
#17019=CARTESIAN_POINT ( 'NONE',  ( -82.40000000000000568, -30.50624999877097210, 96.99999999999998579 ) ) ;
#17020=ADVANCED_FACE ( 'NONE', ( #7369 ), #13227, .T. ) ;
#17022=CARTESIAN_POINT ( 'NONE',  ( -82.39999999999999147, -33.93356250001229313, 103.4641016151377499 ) ) ;
#17025=ADVANCED_FACE ( 'NONE', ( #8925 ), #17226, .T. ) ;
#17036=CARTESIAN_POINT ( 'NONE',  ( -85.15643035624999868, -31.19062499938548783, 98.40857419181659793 ) ) ;
#17042=AXIS2_PLACEMENT_3D ( 'NONE', #5734, #7003, #960 ) ;
#17046=CARTESIAN_POINT ( 'NONE',  ( -79.64356964374999848, -30.92812499938548498, 99.99999999999998579 ) ) ;
#17066=CARTESIAN_POINT ( 'NONE',  ( -82.39999999999999147, -35.23518749875867684, 103.4641016151377499 ) ) ;
#17075=VERTEX_POINT ( 'NONE', #17566 ) ;
#17081=CARTESIAN_POINT ( 'NONE',  ( -83.77821517812500929, -34.26562499938548711, 97.61286128772489690 ) ) ;
#17086=CARTESIAN_POINT ( 'NONE',  ( -83.20384757729334524, -30.93615380933863079, 96.99999999999997158 ) ) ;
#17092=CARTESIAN_POINT ( 'NONE',  ( -82.39999999999999147, -32.30624999877097281, 96.53589838486223584 ) ) ;
#17093=CARTESIAN_POINT ( 'NONE',  ( -83.90000000000000568, -34.06874999877096855, 97.40192378864668399 ) ) ;
#17096=AXIS2_PLACEMENT_3D ( 'NONE', #4918, #5311, #9596 ) ;
#17106=CARTESIAN_POINT ( 'NONE',  ( -82.40000000000000568, -30.00000000000000355, 99.99999999999998579 ) ) ;
#17110=CARTESIAN_POINT ( 'NONE',  ( -79.39999999999999147, -32.00624999877096855, 101.7320508075688537 ) ) ;
#17114=VECTOR ( 'NONE', #7884, 1000.000000000000000 ) ;
#17122=CARTESIAN_POINT ( 'NONE',  ( -83.90000000000000568, -30.37500000000000355, 102.5980762113533018 ) ) ;
#17132=ADVANCED_FACE ( 'NONE', ( #17472 ), #4081, .T. ) ;
#17134=CARTESIAN_POINT ( 'NONE',  ( -85.15643035625001289, -33.40312499938548285, 99.99999999999998579 ) ) ;
#17138=ORIENTED_EDGE ( 'NONE', *, *, #7661, .T. ) ;
#17144=CARTESIAN_POINT ( 'NONE',  ( -82.39999999999999147, -34.19062499938548427, 103.1828516163667899 ) ) ;
#17154=CARTESIAN_POINT ( 'NONE',  ( -79.39999999999999147, -33.33749999999999858, 98.26794919243110371 ) ) ;
#17165=CARTESIAN_POINT ( 'NONE',  ( -85.40000000000000568, -30.40856250001229455, 101.7320508075688679 ) ) ;
#17167=CARTESIAN_POINT ( 'NONE',  ( -85.40000000000000568, -35.37132790096610080, 98.90809659374338025 ) ) ;
#17170=CARTESIAN_POINT ( 'NONE',  ( -82.40000000000000568, -34.55624999877097281, 97.00000000000000000 ) ) ;
#17173=DIRECTION ( 'NONE',  ( 0.000000000000000000, 0.000000000000000000, -1.000000000000000000 ) ) ;
#17182=CARTESIAN_POINT ( 'NONE',  ( -81.02178482187500208, -33.89062499938548711, 97.61286128772489690 ) ) ;
#17191=CARTESIAN_POINT ( 'NONE',  ( -83.20384757729335945, -34.40759618943233988, 102.9999999999999858 ) ) ;
#17192=CARTESIAN_POINT ( 'NONE',  ( -83.90000000000000568, -32.26874999877097139, 97.40192378864668399 ) ) ;
#17193=CARTESIAN_POINT ( 'NONE',  ( -79.64356964375001269, -31.34062499938548640, 98.40857419181659793 ) ) ;
#17205=CARTESIAN_POINT ( 'NONE',  ( -83.77821517812500929, -30.21562499938548285, 97.61286128772489690 ) ) ;
#17215=CARTESIAN_POINT ( 'NONE',  ( -85.40000000000000568, -34.45856250001228460, 101.7320508075688679 ) ) ;
#17218=CARTESIAN_POINT ( 'NONE',  ( -82.39999999999999147, -34.33124999877097139, 103.0000000000000000 ) ) ;
#17219=CARTESIAN_POINT ( 'NONE',  ( -81.59615242270665192, -33.28259618943233278, 97.00000000000000000 ) ) ;
#17226=( BOUNDED_SURFACE ( )  B_SPLINE_SURFACE ( 1, 2, ( 
 ( #15474, #2186, #353, #9312, #16742, #15373, #6299, #3355, #9610, #18409, #1891, #12250, #2086, #13608, #4836, #18218, #10779, #15573, #10969, #12347, #5124, #4738, #6587, #11067, #15276, #17036, #1989, #8042, #3647, #9507, #3551, #536, #12534, #13712, #250, #6207, #16939, #14000, #18506, #7946, #12155, #6492, #10683, #18122, #9210, #16651, #638, #12441, #7849, #3254, #13803, #15176, #1793, #446, #7757, #6393, #13898, #18313, #4932, #5029, #10876, #16847, #3451, #9408, #6971, #18894, #13019, #16050, #12923, #17519, #2557, #18704, #5323, #17428, #14380, #733, #11361, #3740, #9998, #5219, #2471, #3834, #11556, #15954, #17134, #14471, #6881, #12829, #9802, #6787, #14191, #8520, #18796, #1019, #11169, #17230, #5514, #11262, #4132, #7060, #18605, #1102, #9901, #11460, #18991, #5421, #12735, #15864, #8427, #4039, #17326, #15764, #14094, #828, #10092, #2371, #3935, #5612, #8142, #14288, #12631, #6687, #9707, #15668, #2277, #8241, #8332, #924, #2855, #14967, #1303, #8812, #14668, #9006, #7161 ),
 ( #13110, #19177, #4326, #14567, #6085, #4513, #10572, #8714, #17711, #5790, #4418, #7250, #11744, #18003, #7445, #10286, #13205, #10469, #2653, #16246, #14767, #1396, #4616, #34, #7347, #13496, #19080, #1589, #135, #13301, #12032, #10377, #16435, #8616, #17907, #11936, #8902, #7537, #2759, #1204, #5699, #5984, #3044, #11651, #16339, #17611, #14864, #4227, #10183, #16146, #19276, #5892, #11840, #17808, #2948, #1491, #13402, #12485, #589, #18551, #3497, #6539, #12780, #2226, #5076, #9456, #5272, #5368, #7993, #15421, #13949, #18749, #14142, #15521, #8284, #7897, #9752, #14235, #2032, #873, #5166, #11217, #6836, #12677, #6732, #3694, #15716, #16893, #16536, #3136, #776, #18651, #2321, #11113, #9095, #9660, #13847, #15060, #12393, #488, #17182, #15620, #18455, #1936, #11017, #6441, #18361, #16982, #3786, #4983, #17081, #10925, #3594, #8192, #9555, #2138, #8096, #14048, #683, #6635, #12583, #8664, #17372, #14332, #1059, #14425, #17661, #7112, #2511, #10237, #3885, #5655, #8381, #8468, #18845 ) ),
 .UNSPECIFIED., .F., .F., .F. ) 
 B_SPLINE_SURFACE_WITH_KNOTS ( ( 2, 2 ),
 ( 3, 2, 2, 2, 2, 2, 2, 2, 2, 2, 2, 2, 2, 2, 2, 2, 2, 2, 2, 2, 2, 2, 2, 2, 2, 2, 2, 2, 2, 2, 2, 2, 2, 2, 2, 2, 2, 2, 2, 2, 2, 2, 2, 2, 2, 2, 2, 2, 2, 2, 2, 2, 2, 2, 2, 2, 2, 2, 2, 2, 2, 2, 2, 2, 2, 2, 2, 3 ),
 ( 0.000000000000000000, 1.000000000000000000 ),
 ( 0.000000000000000000, 0.01388888888888888812, 0.02777777777777777624, 0.04166666666666666435, 0.05555555555555555247, 0.06944444444444444753, 0.08333333333333332871, 0.09722222222222222376, 0.1111111111111111049, 0.1250000000000000000, 0.1388888888888888951, 0.1527777777777777901, 0.1666666666666666574, 0.1805555555555555525, 0.1944444444444444475, 0.2083333333333333426, 0.2222222222222222099, 0.2361111111111111049, 0.2500000000000000000, 0.2638888888888888951, 0.2777777777777777901, 0.2916666666666666852, 0.3055555555555555802, 0.3194444444444444198, 0.3333333333333333148, 0.3472222222222222099, 0.3611111111111111049, 0.3750000000000000000, 0.3888888888888888951, 0.4027777777777777901, 0.4166666666666666852, 0.4305555555555555802, 0.4444444444444444198, 0.4583333333333333148, 0.4722222222222222099, 0.4861111111111111049, 0.5000000000000000000, 0.5138888888888888395, 0.5277777777777777901, 0.5416666666666666297, 0.5555555555555555802, 0.5694444444444444198, 0.5833333333333333703, 0.5972222222222222099, 0.6111111111111111605, 0.6250000000000000000, 0.6388888888888888395, 0.6527777777777777901, 0.6666666666666666297, 0.6805555555555555802, 0.6944444444444444198, 0.7083333333333333703, 0.7222222222222222099, 0.7361111111111111605, 0.7500000000000000000, 0.7638888888888888395, 0.7777777777777777901, 0.7916666666666666297, 0.8055555555555555802, 0.8194444444444444198, 0.8333333333333333703, 0.8472222222222222099, 0.8611111111111111605, 0.8750000000000000000, 0.8888888888888888395, 0.9027777777777777901, 0.9166666666666666297, 0.9258785565094813652 ),
 .UNSPECIFIED. ) 
 GEOMETRIC_REPRESENTATION_ITEM ( )  RATIONAL_B_SPLINE_SURFACE ( (
 ( 1.000000000000000000, 0.8660254037844387076, 1.000000000000000000, 0.8660254037844387076, 1.000000000000000000, 0.8660254037844387076, 1.000000000000000000, 0.8660254037844387076, 1.000000000000000000, 0.8660254037844387076, 1.000000000000000000, 0.8660254037844387076, 1.000000000000000000, 0.8660254037844387076, 1.000000000000000000, 0.8660254037844387076, 1.000000000000000000, 0.8660254037844387076, 1.000000000000000000, 0.8660254037844387076, 1.000000000000000000, 0.8660254037844387076, 1.000000000000000000, 0.8660254037844387076, 1.000000000000000000, 0.8660254037844387076, 1.000000000000000000, 0.8660254037844387076, 1.000000000000000000, 0.8660254037844387076, 1.000000000000000000, 0.8660254037844387076, 1.000000000000000000, 0.8660254037844387076, 1.000000000000000000, 0.8660254037844387076, 1.000000000000000000, 0.8660254037844387076, 1.000000000000000000, 0.8660254037844387076, 1.000000000000000000, 0.8660254037844387076, 1.000000000000000000, 0.8660254037844387076, 1.000000000000000000, 0.8660254037844387076, 1.000000000000000000, 0.8660254037844387076, 1.000000000000000000, 0.8660254037844387076, 1.000000000000000000, 0.8660254037844387076, 1.000000000000000000, 0.8660254037844387076, 1.000000000000000000, 0.8660254037844387076, 1.000000000000000000, 0.8660254037844387076, 1.000000000000000000, 0.8660254037844387076, 1.000000000000000000, 0.8660254037844387076, 1.000000000000000000, 0.8660254037844387076, 1.000000000000000000, 0.8660254037844387076, 1.000000000000000000, 0.8660254037844387076, 1.000000000000000000, 0.8660254037844387076, 1.000000000000000000, 0.8660254037844387076, 1.000000000000000000, 0.8660254037844387076, 1.000000000000000000, 0.8660254037844387076, 1.000000000000000000, 0.8660254037844387076, 1.000000000000000000, 0.8660254037844387076, 1.000000000000000000, 0.8660254037844387076, 1.000000000000000000, 0.8660254037844387076, 1.000000000000000000, 0.8660254037844387076, 1.000000000000000000, 0.8660254037844387076, 1.000000000000000000, 0.8660254037844387076, 1.000000000000000000, 0.8660254037844387076, 1.000000000000000000, 0.8660254037844387076, 1.000000000000000000, 0.8660254037844387076, 1.000000000000000000, 0.8660254037844387076, 1.000000000000000000, 0.8660254037844387076, 1.000000000000000000, 0.8660254037844387076, 1.000000000000000000, 0.8660254037844387076, 1.000000000000000000, 0.8660254037844387076, 1.000000000000000000, 0.8660254037844387076, 1.000000000000000000, 0.8660254037844387076, 1.000000000000000000, 0.8660254037844387076, 1.000000000000000000, 0.8660254037844387076, 1.000000000000000000, 0.8660254037844387076, 1.000000000000000000, 0.8660254037844387076, 1.000000000000000000, 0.8660254037844387076, 1.000000000000000000, 0.8660254037844387076, 1.000000000000000000, 0.8660254037844387076, 1.000000000000000000, 0.8660254037844387076, 1.000000000000000000, 0.8660254037844387076, 1.000000000000000000, 0.8660254037844387076, 1.000000000000000000, 0.8660254037844387076, 1.000000000000000000, 0.9111405360107203144, 0.9401542295229963209),
 ( 1.000000000000000000, 0.8660254037844387076, 1.000000000000000000, 0.8660254037844387076, 1.000000000000000000, 0.8660254037844387076, 1.000000000000000000, 0.8660254037844387076, 1.000000000000000000, 0.8660254037844387076, 1.000000000000000000, 0.8660254037844387076, 1.000000000000000000, 0.8660254037844387076, 1.000000000000000000, 0.8660254037844387076, 1.000000000000000000, 0.8660254037844387076, 1.000000000000000000, 0.8660254037844387076, 1.000000000000000000, 0.8660254037844387076, 1.000000000000000000, 0.8660254037844387076, 1.000000000000000000, 0.8660254037844387076, 1.000000000000000000, 0.8660254037844387076, 1.000000000000000000, 0.8660254037844387076, 1.000000000000000000, 0.8660254037844387076, 1.000000000000000000, 0.8660254037844387076, 1.000000000000000000, 0.8660254037844387076, 1.000000000000000000, 0.8660254037844387076, 1.000000000000000000, 0.8660254037844387076, 1.000000000000000000, 0.8660254037844387076, 1.000000000000000000, 0.8660254037844387076, 1.000000000000000000, 0.8660254037844387076, 1.000000000000000000, 0.8660254037844387076, 1.000000000000000000, 0.8660254037844387076, 1.000000000000000000, 0.8660254037844387076, 1.000000000000000000, 0.8660254037844387076, 1.000000000000000000, 0.8660254037844387076, 1.000000000000000000, 0.8660254037844387076, 1.000000000000000000, 0.8660254037844387076, 1.000000000000000000, 0.8660254037844387076, 1.000000000000000000, 0.8660254037844387076, 1.000000000000000000, 0.8660254037844387076, 1.000000000000000000, 0.8660254037844387076, 1.000000000000000000, 0.8660254037844387076, 1.000000000000000000, 0.8660254037844387076, 1.000000000000000000, 0.8660254037844387076, 1.000000000000000000, 0.8660254037844387076, 1.000000000000000000, 0.8660254037844387076, 1.000000000000000000, 0.8660254037844387076, 1.000000000000000000, 0.8660254037844387076, 1.000000000000000000, 0.8660254037844387076, 1.000000000000000000, 0.8660254037844387076, 1.000000000000000000, 0.8660254037844387076, 1.000000000000000000, 0.8660254037844387076, 1.000000000000000000, 0.8660254037844387076, 1.000000000000000000, 0.8660254037844387076, 1.000000000000000000, 0.8660254037844387076, 1.000000000000000000, 0.8660254037844387076, 1.000000000000000000, 0.8660254037844387076, 1.000000000000000000, 0.8660254037844387076, 1.000000000000000000, 0.8660254037844387076, 1.000000000000000000, 0.8660254037844387076, 1.000000000000000000, 0.8660254037844387076, 1.000000000000000000, 0.8660254037844387076, 1.000000000000000000, 0.8660254037844387076, 1.000000000000000000, 0.8660254037844387076, 1.000000000000000000, 0.8660254037844387076, 1.000000000000000000, 0.8660254037844387076, 1.000000000000000000, 0.8660254037844387076, 1.000000000000000000, 0.8660254037844387076, 1.000000000000000000, 0.8660254037844387076, 1.000000000000000000, 0.8660254037844387076, 1.000000000000000000, 0.8660254037844387076, 1.000000000000000000, 0.8660254037844387076, 1.000000000000000000, 0.8660254037844387076, 1.000000000000000000, 0.9111405360107203144, 0.9401542295229963209) ) ) 
 REPRESENTATION_ITEM ( '' )  SURFACE ( )  );
#17230=CARTESIAN_POINT ( 'NONE',  ( -85.15643035624999868, -33.81562499938549138, 101.5914258081833879 ) ) ;
#17234=CARTESIAN_POINT ( 'NONE',  ( -81.02178482187500208, -34.49062499938548854, 102.3871387122750889 ) ) ;
#17242=CARTESIAN_POINT ( 'NONE',  ( -79.64356964374999848, -34.07812499938548711, 99.99999999999998579 ) ) ;
#17250=VERTEX_POINT ( 'NONE', #322 ) ;
#17253=CARTESIAN_POINT ( 'NONE',  ( -82.39999999999999147, -34.38750000000000284, 103.4641016151377499 ) ) ;
#17259=ORIENTED_EDGE ( 'NONE', *, *, #11875, .T. ) ;
#17291=CARTESIAN_POINT ( 'NONE',  ( -83.90000000000000568, -34.36874999877097281, 102.5980762113533018 ) ) ;
#17292=CARTESIAN_POINT ( 'NONE',  ( -85.15643035625001289, -32.05312499938548854, 99.99999999999998579 ) ) ;
#17303=CARTESIAN_POINT ( 'NONE',  ( -81.02178482187500208, -31.64062499938548356, 97.61286128772489690 ) ) ;
#17314=CARTESIAN_POINT ( 'NONE',  ( -83.90000000000000568, -34.87106250001230023, 102.5980762113533018 ) ) ;
#17326=CARTESIAN_POINT ( 'NONE',  ( -83.77821517812500929, -34.37812499938548427, 97.61286128772489690 ) ) ;
#17330=CARTESIAN_POINT ( 'NONE',  ( -85.15643035624999868, -32.87812499938549138, 98.40857419181659793 ) ) ;
#17337=CARTESIAN_POINT ( 'NONE',  ( -82.39999999999999147, -33.96562499938548285, 96.81714838363319586 ) ) ;
#17348=CARTESIAN_POINT ( 'NONE',  ( -85.40000000000000568, -33.14999999999999858, 99.99999999999998579 ) ) ;
#17355=CARTESIAN_POINT ( 'NONE',  ( -79.39999999999999147, -31.15856250001229455, 101.7320508075688537 ) ) ;
#17360=CARTESIAN_POINT ( 'NONE',  ( -85.15643035624999868, -30.55312499938548854, 101.5914258081833879 ) ) ;
#17372=CARTESIAN_POINT ( 'NONE',  ( -83.77821517812500929, -34.71562499938548285, 97.61286128772489690 ) ) ;
#17383=CARTESIAN_POINT ( 'NONE',  ( -80.90000000000000568, -33.84374999877096712, 102.5980762113533018 ) ) ;
#17385=CARTESIAN_POINT ( 'NONE',  ( -83.77821517812500929, -31.67812499938548498, 97.61286128772489690 ) ) ;
#17387=( BOUNDED_CURVE ( )  B_SPLINE_CURVE ( 2, ( #14189, #12532, #1889, #12629, #8040, #3549, #6685, #16845, #10968 ),
 .UNSPECIFIED., .F., .F. ) 
 B_SPLINE_CURVE_WITH_KNOTS ( ( 3, 2, 2, 2, 3 ),
 ( 0.6458333333333333703, 0.6527777777777777901, 0.6666666666666666297, 0.6805555555555555802, 0.6875000000000000000 ),
 .UNSPECIFIED. ) 
 CURVE ( )  GEOMETRIC_REPRESENTATION_ITEM ( )  RATIONAL_B_SPLINE_CURVE ( ( 0.9330127018922192983, 0.9330127018922198534, 1.000000000000000000, 0.8660254037844387076, 1.000000000000000000, 0.8660254037844387076, 1.000000000000000000, 0.9330127018922194093, 0.9330127018922194093 ) ) 
 REPRESENTATION_ITEM ( '' )  );
#17393=ORIENTED_EDGE ( 'NONE', *, *, #7314, .F. ) ;
#17398=CARTESIAN_POINT ( 'NONE',  ( -79.39999999999999147, -35.08124999877097139, 98.26794919243110371 ) ) ;
#17399=CARTESIAN_POINT ( 'NONE',  ( -79.64356964374998427, -30.40312499938548285, 101.5914258081833879 ) ) ;
#17405=ORIENTED_EDGE ( 'NONE', *, *, #5561, .T. ) ;
#17412=CARTESIAN_POINT ( 'NONE',  ( -79.39999999999999147, -31.16250000000000497, 101.7320508075688537 ) ) ;
#17428=CARTESIAN_POINT ( 'NONE',  ( -85.15643035624999868, -32.99062499938548854, 98.40857419181659793 ) ) ;
#17432=CARTESIAN_POINT ( 'NONE',  ( -81.02178482187500208, -33.14062499938548711, 102.3871387122750889 ) ) ;
#17436=AXIS2_PLACEMENT_3D ( 'NONE', #11255, #724, #15755 ) ;
#17438=CARTESIAN_POINT ( 'NONE',  ( -85.15643035625001289, -32.91562499938548569, 101.5914258081833879 ) ) ;
#17448=CARTESIAN_POINT ( 'NONE',  ( -85.40000000000000568, -32.73750000000000426, 98.26794919243111792 ) ) ;
#17455=CARTESIAN_POINT ( 'NONE',  ( -82.39999999999999147, -31.23356250001229384, 103.4641016151377499 ) ) ;
#17470=ADVANCED_FACE ( 'NONE', ( #14855 ), #7338, .T. ) ;
#17472=FACE_OUTER_BOUND ( 'NONE', #14910, .T. ) ;
#17481=CARTESIAN_POINT ( 'NONE',  ( -83.20384757729338787, -34.59240381056766722, 97.00000000000000000 ) ) ;
#17482=CARTESIAN_POINT ( 'NONE',  ( -85.40000000000000568, -34.44374999877096855, 99.99999999999998579 ) ) ;
#17483=CARTESIAN_POINT ( 'NONE',  ( -85.15643035624999868, -31.11562499938548854, 101.5914258081833879 ) ) ;
#17486=EDGE_CURVE ( 'NONE', #10662, #14886, #7309, .T. ) ;
#17491=ORIENTED_EDGE ( 'NONE', *, *, #10075, .T. ) ;
#17495=CARTESIAN_POINT ( 'NONE',  ( -84.69814161231455785, -35.39427329483935836, 98.07164704222790874 ) ) ;
#17506=CARTESIAN_POINT ( 'NONE',  ( -80.90000000000000568, -31.50000000000000000, 97.40192378864668399 ) ) ;
#17512=( BOUNDED_CURVE ( )  B_SPLINE_CURVE ( 1, ( #17601, #4214 ),
 .UNSPECIFIED., .F., .F. ) 
 B_SPLINE_CURVE_WITH_KNOTS ( ( 2, 2 ),
 ( 0.000000000000000000, 1.000000000000000000 ),
 .UNSPECIFIED. ) 
 CURVE ( )  GEOMETRIC_REPRESENTATION_ITEM ( )  RATIONAL_B_SPLINE_CURVE ( ( 0.9401539157124900736, 0.9401539157124900736 ) ) 
 REPRESENTATION_ITEM ( '' )  );
#17513=CARTESIAN_POINT ( 'NONE',  ( -81.59615242270662350, -31.03259618943233988, 96.99999999999998579 ) ) ;
#17519=CARTESIAN_POINT ( 'NONE',  ( -82.39999999999999147, -32.84062499938548996, 103.1828516163667899 ) ) ;
#17524=CARTESIAN_POINT ( 'NONE',  ( -85.15643035625001289, -32.84062499938548285, 99.99999999999998579 ) ) ;
#17525=DIRECTION ( 'NONE',  ( -0.000000000000000000, -1.000000000000000000, -0.000000000000000000 ) ) ;
#17540=CARTESIAN_POINT ( 'NONE',  ( -82.39999999999999147, -33.93750000000000000, 103.4641016151377499 ) ) ;
#17544=CARTESIAN_POINT ( 'NONE',  ( -83.90000000000000568, -30.52500000000000213, 97.40192378864668399 ) ) ;
#17552=CARTESIAN_POINT ( 'NONE',  ( -79.64356964375001269, -30.40312499938548285, 101.5914258081833879 ) ) ;
#17566=CARTESIAN_POINT ( 'NONE',  ( -85.40000000000000568, -30.39374999877097139, 99.99999999999998579 ) ) ;
#17572=APPLICATION_CONTEXT ( 'automotive_design' ) ;
#17577=CARTESIAN_POINT ( 'NONE',  ( -79.39999999999999147, -34.66874999877096997, 99.99999999999998579 ) ) ;
#17578=CARTESIAN_POINT ( 'NONE',  ( -82.39999999999999147, -31.04062499938548569, 103.1828516163667899 ) ) ;
#17579=CARTESIAN_POINT ( 'NONE',  ( -80.90000000000000568, -30.69374999877097210, 102.5980762113533018 ) ) ;
#17588=CARTESIAN_POINT ( 'NONE',  ( -82.39999999999999147, -32.05312499938548854, 96.81714838363319586 ) ) ;
#17599=CARTESIAN_POINT ( 'NONE',  ( -83.90000000000000568, -32.17500000000000426, 102.5980762113533018 ) ) ;
#17601=CARTESIAN_POINT ( 'NONE',  ( -84.70833260042415702, -35.00006955123599539, 98.08383195543535749 ) ) ;
#17611=CARTESIAN_POINT ( 'NONE',  ( -82.39999999999999147, -31.82812499938548356, 103.1828516163667899 ) ) ;
#17618=CARTESIAN_POINT ( 'NONE',  ( -85.15643035624999868, -34.60312499938548569, 101.5914258081833879 ) ) ;
#17645=CARTESIAN_POINT ( 'NONE',  ( -85.40000000000000568, -33.55856250001229313, 101.7320508075688679 ) ) ;
#17649=CARTESIAN_POINT ( 'NONE',  ( -85.15643035625001289, -31.49062499938548498, 99.99999999999998579 ) ) ;
#17650=CARTESIAN_POINT ( 'NONE',  ( -83.90000000000000568, -32.71874999877096712, 97.40192378864668399 ) ) ;
#17661=CARTESIAN_POINT ( 'NONE',  ( -79.64356964374999848, -34.86562499938548143, 99.99999999999998579 ) ) ;
#17672=CARTESIAN_POINT ( 'NONE',  ( -85.40000000000000568, -34.85624999877096997, 101.7320508075688679 ) ) ;
#17673=CARTESIAN_POINT ( 'NONE',  ( -82.39999999999999147, -33.96562499938548285, 96.81714838363319586 ) ) ;
#17676=CARTESIAN_POINT ( 'NONE',  ( -82.40000000000000568, -30.00000000000000355, 103.0000000000000000 ) ) ;
#17685=CARTESIAN_POINT ( 'NONE',  ( -85.15643035625001289, -32.87812499938548427, 98.40857419181659793 ) ) ;
#17697=CARTESIAN_POINT ( 'NONE',  ( -83.90000000000000568, -32.62500000000000000, 102.5980762113533018 ) ) ;
#17711=CARTESIAN_POINT ( 'NONE',  ( -81.02178482187500208, -30.44062499938548783, 102.3871387122750889 ) ) ;
#17714=AXIS2_PLACEMENT_3D ( 'NONE', #5935, #14867, #3179 ) ;
#17720=CARTESIAN_POINT ( 'NONE',  ( -85.40000000000000568, -31.83750000000000568, 98.26794919243111792 ) ) ;
#17721=CARTESIAN_POINT ( 'NONE',  ( -79.39999999999999147, -32.06250000000000000, 101.7320508075688537 ) ) ;
#17728=CARTESIAN_POINT ( 'NONE',  ( -85.15643035625001289, -35.20312499938548711, 99.99999999999998579 ) ) ;
#17750=CARTESIAN_POINT ( 'NONE',  ( -83.90000000000000568, -31.87106250001229313, 97.40192378864668399 ) ) ;
#17753=CARTESIAN_POINT ( 'NONE',  ( -81.02178482187500208, -31.79062499938548925, 102.3871387122750889 ) ) ;
#17775=CARTESIAN_POINT ( 'NONE',  ( -79.39999999999999147, -32.38518749875867542, 98.26794919243110371 ) ) ;
#17776=CARTESIAN_POINT ( 'NONE',  ( -83.77821517812500929, -33.77812499938548285, 102.3871387122750889 ) ) ;
#17787=CARTESIAN_POINT ( 'NONE',  ( -83.77821517812500929, -33.21562499938548285, 102.3871387122750889 ) ) ;
#17796=CARTESIAN_POINT ( 'NONE',  ( -82.39999999999999147, -33.03750000000000142, 103.4641016151377499 ) ) ;
#17797=CARTESIAN_POINT ( 'NONE',  ( -85.40000000000000568, -31.74374999877096926, 99.99999999999998579 ) ) ;
#17808=CARTESIAN_POINT ( 'NONE',  ( -79.64356964375001269, -32.12812499938548427, 98.40857419181659793 ) ) ;
#17813=CARTESIAN_POINT ( 'NONE',  ( -83.20384757729337366, -31.70759618943234059, 103.0000000000000000 ) ) ;
#17814=CARTESIAN_POINT ( 'NONE',  ( -83.88339518848731302, -35.16733441503058089, 97.47959136244114120 ) ) ;
#17826=ORIENTED_EDGE ( 'NONE', *, *, #2937, .T. ) ;
#17834=CARTESIAN_POINT ( 'NONE',  ( -80.90000000000000568, -30.99374999877096926, 97.40192378864668399 ) ) ;
#17836=CARTESIAN_POINT ( 'NONE',  ( -80.90000000000000568, -33.44606250001229597, 102.5980762113533018 ) ) ;
#17839=CARTESIAN_POINT ( 'NONE',  ( -81.02178482187500208, -30.89062499938548711, 102.3871387122750889 ) ) ;
#17857=EDGE_LOOP ( 'NONE', ( #18023, #1615, #14993, #2600 ) ) ;
#17866=CARTESIAN_POINT ( 'NONE',  ( -80.90000000000000568, -31.44768749875867542, 97.40192378864668399 ) ) ;
#17867=CARTESIAN_POINT ( 'NONE',  ( -85.15643035625001289, -33.85312499938549280, 99.99999999999998579 ) ) ;
#17882=CARTESIAN_POINT ( 'NONE',  ( -83.77821517812500929, -34.56562499938548427, 102.3871387122750889 ) ) ;
#17893=CARTESIAN_POINT ( 'NONE',  ( -85.40000000000000568, -34.08749999999999858, 98.26794919243111792 ) ) ;
#17894=CARTESIAN_POINT ( 'NONE',  ( -85.40000000000000568, -31.78124999877096712, 98.26794919243111792 ) ) ;
#17903=FACE_OUTER_BOUND ( 'NONE', #16830, .T. ) ;
#17907=CARTESIAN_POINT ( 'NONE',  ( -83.77821517812500929, -31.41562499938548569, 102.3871387122750889 ) ) ;
#17910=ORIENTED_EDGE ( 'NONE', *, *, #16871, .F. ) ;
#17913=CARTESIAN_POINT ( 'NONE',  ( -85.40000000000000568, -30.41249999999999787, 101.7320508075688679 ) ) ;
#17921=ORIENTED_EDGE ( 'NONE', *, *, #9148, .T. ) ;
#17931=( BOUNDED_CURVE ( )  B_SPLINE_CURVE ( 2, ( #10691, #18319, #16658, #7475, #11962, #9127, #3260, #1897, #4745 ),
 .UNSPECIFIED., .F., .F. ) 
 B_SPLINE_CURVE_WITH_KNOTS ( ( 3, 2, 2, 2, 3 ),
 ( 0.4375000000000000555, 0.4444444444444444198, 0.4583333333333333148, 0.4722222222222222099, 0.4791666666666666297 ),
 .UNSPECIFIED. ) 
 CURVE ( )  GEOMETRIC_REPRESENTATION_ITEM ( )  RATIONAL_B_SPLINE_CURVE ( ( 0.9330127018922192983, 0.9330127018922198534, 1.000000000000000000, 0.8660254037844387076, 1.000000000000000000, 0.8660254037844387076, 1.000000000000000000, 0.9330127018922196314, 0.9330127018922194093 ) ) 
 REPRESENTATION_ITEM ( '' )  );
#17934=CARTESIAN_POINT ( 'NONE',  ( -79.39999999999999147, -31.98356250001229384, 98.26794919243110371 ) ) ;
#17937=CARTESIAN_POINT ( 'NONE',  ( -82.39999999999999147, -32.05312499938548854, 96.81714838363319586 ) ) ;
#17941=FACE_OUTER_BOUND ( 'NONE', #3554, .T. ) ;
#17950=CARTESIAN_POINT ( 'NONE',  ( -85.40000000000000568, -33.14999999999999858, 99.99999999999998579 ) ) ;
#17961=CARTESIAN_POINT ( 'NONE',  ( -80.90000000000000568, -32.34768749875867400, 97.40192378864668399 ) ) ;
#17962=CARTESIAN_POINT ( 'NONE',  ( -83.77821517812500929, -34.67812499938548854, 102.3871387122750889 ) ) ;
#17978=CARTESIAN_POINT ( 'NONE',  ( -83.77821517812500929, -32.46562499938548285, 97.61286128772489690 ) ) ;
#17985=EDGE_LOOP ( 'NONE', ( #16068, #12513, #15469, #15568 ) ) ;
#17989=CARTESIAN_POINT ( 'NONE',  ( -85.40000000000000568, -33.60000000000000142, 99.99999999999998579 ) ) ;
#17990=CARTESIAN_POINT ( 'NONE',  ( -79.39999999999999147, -31.06874999877096855, 99.99999999999998579 ) ) ;
#18003=CARTESIAN_POINT ( 'NONE',  ( -85.15643035624999868, -30.62812499938548427, 98.40857419181659793 ) ) ;
#18008=ORIENTED_EDGE ( 'NONE', *, *, #555, .T. ) ;
#18011=CARTESIAN_POINT ( 'NONE',  ( -83.25523545990762386, -35.19352049914630953, 96.73097394877602540 ) ) ;
#18023=ORIENTED_EDGE ( 'NONE', *, *, #13688, .F. ) ;
#18031=CARTESIAN_POINT ( 'NONE',  ( -79.39999999999999147, -34.76250000000000284, 101.7320508075688537 ) ) ;
#18035=VECTOR ( 'NONE', #329, 1000.000000000000000 ) ;
#18038=CARTESIAN_POINT ( 'NONE',  ( -80.90000000000000568, -32.99606250001229313, 102.5980762113533018 ) ) ;
#18050=ORIENTED_EDGE ( 'NONE', *, *, #2229, .T. ) ;
#18063=CARTESIAN_POINT ( 'NONE',  ( -79.39999999999999147, -32.87268749875867968, 99.99999999999998579 ) ) ;
#18064=CARTESIAN_POINT ( 'NONE',  ( -81.02178482187500208, -34.15312499938548285, 102.3871387122750889 ) ) ;
#18078=CARTESIAN_POINT ( 'NONE',  ( -82.39999999999999147, -33.62812499938548427, 103.1828516163667899 ) ) ;
#18085=FACE_OUTER_BOUND ( 'NONE', #9293, .T. ) ;
#18089=CARTESIAN_POINT ( 'NONE',  ( -79.39999999999999147, -30.58124999877096784, 98.26794919243110371 ) ) ;
#18090=CARTESIAN_POINT ( 'NONE',  ( -83.90000000000000568, -31.36874999877096926, 97.40192378864668399 ) ) ;
#18104=FACE_BOUND ( 'NONE', #6088, .T. ) ;
#18109=CARTESIAN_POINT ( 'NONE',  ( -82.39999999999999147, -30.56250000000000355, 96.53589838486223584 ) ) ;
#18121=CARTESIAN_POINT ( 'NONE',  ( -82.39999999999999147, -32.98124999877096286, 102.9999999999999858 ) ) ;
#18122=CARTESIAN_POINT ( 'NONE',  ( -79.64356964375001269, -31.86562499938548143, 101.5914258081833879 ) ) ;
#18127=CARTESIAN_POINT ( 'NONE',  ( -79.77381699087979428, -34.99985067802517591, 101.4917037897926093 ) ) ;
#18129=CARTESIAN_POINT ( 'NONE',  ( -85.40000000000000568, -30.86250000000000071, 101.7320508075688679 ) ) ;
#18131=CARTESIAN_POINT ( 'NONE',  ( -81.02178482187500208, -32.20312499938548711, 97.61286128772489690 ) ) ;
#18153=CARTESIAN_POINT ( 'NONE',  ( -82.39999999999999147, -31.86018749875867684, 96.53589838486223584 ) ) ;
#18162=AXIS2_PLACEMENT_3D ( 'NONE', #6564, #15742, #11242 ) ;
#18180=CARTESIAN_POINT ( 'NONE',  ( -82.39999999999999147, -30.50624999877097210, 96.53589838486223584 ) ) ;
#18181=CARTESIAN_POINT ( 'NONE',  ( -82.39999999999999147, -31.63124999877097210, 103.4641016151377499 ) ) ;
#18189=SURFACE_SIDE_STYLE ('',( #15342 ) ) ;
#18194=ORIENTED_EDGE ( 'NONE', *, *, #2354, .F. ) ;
#18218=CARTESIAN_POINT ( 'NONE',  ( -82.39999999999999147, -30.81562499938548427, 96.81714838363319586 ) ) ;
#18224=CARTESIAN_POINT ( 'NONE',  ( -79.39999999999999147, -31.06874999877096855, 99.99999999999998579 ) ) ;
#18227=ADVANCED_FACE ( 'NONE', ( #10769 ), #4633, .T. ) ;
#18228=CARTESIAN_POINT ( 'NONE',  ( -81.02178482187500208, -31.45312499938549067, 102.3871387122750889 ) ) ;
#18235=VERTEX_POINT ( 'NONE', #3058 ) ;
#18249=CARTESIAN_POINT ( 'NONE',  ( -83.90000000000000568, -34.82268749875867542, 102.5980762113533018 ) ) ;
#18256=( BOUNDED_CURVE ( )  B_SPLINE_CURVE ( 2, ( #8693, #11241, #17205, #12804, #2731, #4014, #16124, #17399, #3809, #899, #18868, #15741, #9976, #2347, #16026, #2449, #10067, #14261, #12901, #14448, #13088, #2532, #6859, #8591, #6948, #14643, #14356, #8493, #6761, #18771, #5393, #1179, #12704, #7038, #7137, #3909, #1081, #11338, #15837, #4106, #17303, #8404, #18965, #5587, #11534, #2627, #18677, #19058, #5680, #9876, #11623, #17588, #4200, #10160, #5490, #5295, #11437, #13180, #7225, #8785, #6156, #5961, #17978, #1375, #10637, #6060, #3112, #14740, #12006, #4589, #13274, #7321, #9071, #17685, #1277, #12105, #13562, #10547, #16509, #109, #3018, #10445, #17787, #15035, #1658, #7610, #203, #9168, #19249, #16316, #4394, #19152, #7417, #18078, #10351, #14837, #4686, #5765, #10262, #1463, #16603, #8976, #2926, #3209, #11717, #12, #4298, #16225, #13378, #2831, #7513, #5866, #11818, #16409, #8878, #11909, #1567, #14942, #17882, #4490, #13470, #9263, #9360, #4984, #7803, #13950, #16983, #14049, #3406, #12299, #3304, #304, #1845, #11114, #6253 ),
 .UNSPECIFIED., .F., .F. ) 
 B_SPLINE_CURVE_WITH_KNOTS ( ( 3, 2, 2, 2, 2, 2, 2, 2, 2, 2, 2, 2, 2, 2, 2, 2, 2, 2, 2, 2, 2, 2, 2, 2, 2, 2, 2, 2, 2, 2, 2, 2, 2, 2, 2, 2, 2, 2, 2, 2, 2, 2, 2, 2, 2, 2, 2, 2, 2, 2, 2, 2, 2, 2, 2, 2, 2, 2, 2, 2, 2, 2, 2, 2, 2, 2, 2, 3 ),
 ( 0.000000000000000000, 0.01500076742380701197, 0.03000153484761402395, 0.04500230227142103939, 0.06000306969522804790, 0.07500383711903506334, 0.09000460454284207878, 0.1050053719666490942, 0.1200061393904560958, 0.1350069068142631112, 0.1500076742380701267, 0.1650084416618771699, 0.1800092090856841576, 0.1950099765094911730, 0.2100107439332981885, 0.2250115113571052039, 0.2400122787809121916, 0.2550130462047192070, 0.2700138136285262225, 0.2850145810523332379, 0.3000153484761402534, 0.3150161158999473243, 0.3300168833237543398, 0.3450176507475612997, 0.3600184181713683151, 0.3750191855951753306, 0.3900199530189823460, 0.4050207204427893615, 0.4200214878665963769, 0.4350222552904033924, 0.4500230227142104078, 0.4650237901380174232, 0.4800245575618243832, 0.4950253249856313986, 0.5100260924094384141, 0.5250268598332454850, 0.5400276272570524450, 0.5550283946808594049, 0.5700291621046664758, 0.5850299295284734358, 0.6000306969522805067, 0.6150314643760874667, 0.6300322317998946486, 0.6450329992237016086, 0.6600337666475086795, 0.6750345340713156395, 0.6900353014951225994, 0.7050360689189296703, 0.7200368363427366303, 0.7350376037665437012, 0.7500383711903506612, 0.7650391386141577321, 0.7800399060379646921, 0.7950406734617717630, 0.8100414408855787229, 0.8250422083093856829, 0.8400429757331927538, 0.8550437431569997138, 0.8700445105808067847, 0.8850452780046137446, 0.9000460454284208156, 0.9150468128522277755, 0.9300475802760348465, 0.9450483476998418064, 0.9600491151236487664, 0.9750498825474558373, 0.9900506499712627972, 1.000000000000000000 ),
 .UNSPECIFIED. ) 
 CURVE ( )  GEOMETRIC_REPRESENTATION_ITEM ( )  RATIONAL_B_SPLINE_CURVE ( ( 1.000000000000000000, 0.8660254037844387076, 1.000000000000000000, 0.8660254037844387076, 1.000000000000000000, 0.8660254037844387076, 1.000000000000000000, 0.8660254037844387076, 1.000000000000000000, 0.8660254037844387076, 1.000000000000000000, 0.8660254037844387076, 1.000000000000000000, 0.8660254037844387076, 1.000000000000000000, 0.8660254037844387076, 1.000000000000000000, 0.8660254037844387076, 1.000000000000000000, 0.8660254037844387076, 1.000000000000000000, 0.8660254037844387076, 1.000000000000000000, 0.8660254037844387076, 1.000000000000000000, 0.8660254037844387076, 1.000000000000000000, 0.8660254037844387076, 1.000000000000000000, 0.8660254037844387076, 1.000000000000000000, 0.8660254037844387076, 1.000000000000000000, 0.8660254037844387076, 1.000000000000000000, 0.8660254037844387076, 1.000000000000000000, 0.8660254037844387076, 1.000000000000000000, 0.8660254037844387076, 1.000000000000000000, 0.8660254037844387076, 1.000000000000000000, 0.8660254037844387076, 1.000000000000000000, 0.8660254037844387076, 1.000000000000000000, 0.8660254037844387076, 1.000000000000000000, 0.8660254037844387076, 1.000000000000000000, 0.8660254037844387076, 1.000000000000000000, 0.8660254037844387076, 1.000000000000000000, 0.8660254037844387076, 1.000000000000000000, 0.8660254037844387076, 1.000000000000000000, 0.8660254037844387076, 1.000000000000000000, 0.8660254037844387076, 1.000000000000000000, 0.8660254037844387076, 1.000000000000000000, 0.8660254037844387076, 1.000000000000000000, 0.8660254037844387076, 1.000000000000000000, 0.8660254037844387076, 1.000000000000000000, 0.8660254037844387076, 1.000000000000000000, 0.8660254037844387076, 1.000000000000000000, 0.8660254037844387076, 1.000000000000000000, 0.8660254037844387076, 1.000000000000000000, 0.8660254037844387076, 1.000000000000000000, 0.8660254037844387076, 1.000000000000000000, 0.8660254037844387076, 1.000000000000000000, 0.8660254037844387076, 1.000000000000000000, 0.8660254037844387076, 1.000000000000000000, 0.8660254037844387076, 1.000000000000000000, 0.8660254037844387076, 1.000000000000000000, 0.8660254037844387076, 1.000000000000000000, 0.8660254037844387076, 1.000000000000000000, 0.8660254037844387076, 1.000000000000000000, 0.8660254037844387076, 1.000000000000000000, 0.8660254037844387076, 1.000000000000000000, 0.8660254037844387076, 1.000000000000000000, 0.8660254037844387076, 1.000000000000000000, 0.8660254037844387076, 1.000000000000000000, 0.8660254037844387076, 1.000000000000000000, 0.8660254037844387076, 1.000000000000000000, 0.8660254037844387076, 1.000000000000000000, 0.8660254037844387076, 1.000000000000000000, 0.8660254037844387076, 1.000000000000000000, 0.8660254037844387076, 1.000000000000000000, 0.8660254037844387076, 1.000000000000000000, 0.8660254037844387076, 1.000000000000000000, 0.8660254037844387076, 1.000000000000000000, 0.8660254037844387076, 1.000000000000000000, 0.8660254037844387076, 1.000000000000000000, 0.8660254037844387076, 1.000000000000000000, 0.9111405360107203144, 0.9401542295229963209 ) ) 
 REPRESENTATION_ITEM ( '' )  );
#18269=CARTESIAN_POINT ( 'NONE',  ( -82.40000000000000568, -30.00000000000000355, 99.99999999999998579 ) ) ;
#18276=CARTESIAN_POINT ( 'NONE',  ( -83.90000000000000568, -34.42500000000000426, 102.5980762113533018 ) ) ;
#18277=CARTESIAN_POINT ( 'NONE',  ( -80.90000000000000568, -34.74374999877097281, 102.5980762113533018 ) ) ;
#18313=CARTESIAN_POINT ( 'NONE',  ( -82.39999999999999147, -32.39062499938548001, 103.1828516163667899 ) ) ;
#18319=CARTESIAN_POINT ( 'NONE',  ( -81.59615242270662350, -32.38259618943233420, 96.99999999999998579 ) ) ;
#18324=CARTESIAN_POINT ( 'NONE',  ( -81.02178482187500208, -30.40312499938548640, 97.61286128772489690 ) ) ;
#18346=CARTESIAN_POINT ( 'NONE',  ( -83.90000000000000568, -33.92268749875866973, 102.5980762113533018 ) ) ;
#18361=CARTESIAN_POINT ( 'NONE',  ( -83.77821517812500929, -34.11562499938548854, 102.3871387122750889 ) ) ;
#18366=ORIENTED_EDGE ( 'NONE', *, *, #14324, .F. ) ;
#18376=CARTESIAN_POINT ( 'NONE',  ( -82.39999999999999147, -31.18124999877096926, 103.4641016151377499 ) ) ;
#18377=CARTESIAN_POINT ( 'NONE',  ( -83.90000000000000568, -33.61874999877097281, 97.40192378864668399 ) ) ;
#18388=UNCERTAINTY_MEASURE_WITH_UNIT (LENGTH_MEASURE( 1.000000000000000082E-05 ), #5002, 'distance_accuracy_value', 'NONE');
#18400=ADVANCED_FACE ( 'NONE', ( #14182 ), #915, .T. ) ;
#18409=CARTESIAN_POINT ( 'NONE',  ( -82.39999999999999147, -30.59062499938548640, 103.1828516163667899 ) ) ;
#18417=CARTESIAN_POINT ( 'NONE',  ( -83.77821517812500929, -31.67812499938548498, 97.61286128772489690 ) ) ;
#18429=EDGE_CURVE ( 'NONE', #19060, #4909, #10374, .T. ) ;
#18440=CARTESIAN_POINT ( 'NONE',  ( -79.39999999999999147, -33.28518749875868110, 98.26794919243110371 ) ) ;
#18442=CARTESIAN_POINT ( 'NONE',  ( -85.15643035625001289, -35.22676544108147567, 98.99674642581742035 ) ) ;
#18455=CARTESIAN_POINT ( 'NONE',  ( -79.64356964374999848, -33.96562499938548285, 99.99999999999998579 ) ) ;
#18458=ORIENTED_EDGE ( 'NONE', *, *, #4260, .T. ) ;
#18461=FACE_OUTER_BOUND ( 'NONE', #13466, .T. ) ;
#18464=CARTESIAN_POINT ( 'NONE',  ( -82.40000000000000568, -50.00000000000000000, 99.99999999999998579 ) ) ;
#18467=CARTESIAN_POINT ( 'NONE',  ( -79.39999999999999147, -32.45624999877097139, 101.7320508075688537 ) ) ;
#18468=CARTESIAN_POINT ( 'NONE',  ( -79.39999999999999147, -34.70624999877097139, 101.7320508075688537 ) ) ;
#18469=CARTESIAN_POINT ( 'NONE',  ( -82.40000000000001990, -32.13750000000000284, 103.0000000000000000 ) ) ;
#18486=ORIENTED_EDGE ( 'NONE', *, *, #1511, .T. ) ;
#18492=CARTESIAN_POINT ( 'NONE',  ( -85.40000000000000568, -34.90856250001228744, 101.7320508075688679 ) ) ;
#18498=VECTOR ( 'NONE', #14954, 1000.000000000000000 ) ;
#18506=CARTESIAN_POINT ( 'NONE',  ( -83.77821517812500929, -31.67812499938548498, 97.61286128772489690 ) ) ;
#18515=CARTESIAN_POINT ( 'NONE',  ( -85.15643035625001289, -31.60312499938548569, 99.99999999999998579 ) ) ;
#18535=CARTESIAN_POINT ( 'NONE',  ( -82.39999999999999147, -33.88518749875868252, 103.4641016151377499 ) ) ;
#18537=CARTESIAN_POINT ( 'NONE',  ( -81.02178482187500208, -34.90312499938548285, 97.61286128772489690 ) ) ;
#18538=DIRECTION ( 'NONE',  ( 0.000000000000000000, -1.000000000000000000, 0.000000000000000000 ) ) ;
#18551=CARTESIAN_POINT ( 'NONE',  ( -85.15643035624999868, -32.35312499938549280, 101.5914258081833879 ) ) ;
#18561=CARTESIAN_POINT ( 'NONE',  ( -82.39999999999999147, -31.91249999999999787, 96.99999999999998579 ) ) ;
#18562=CARTESIAN_POINT ( 'NONE',  ( -79.39999999999999147, -31.55624999877096926, 101.7320508075688537 ) ) ;
#18563=CARTESIAN_POINT ( 'NONE',  ( -79.39999999999999147, -34.18124999877097281, 98.26794919243110371 ) ) ;
#18564=CARTESIAN_POINT ( 'NONE',  ( -85.40000000000000568, -32.21250000000000568, 101.7320508075688821 ) ) ;
#18578=ADVANCED_BREP_SHAPE_REPRESENTATION ( '', ( #9467, #10540 ), #9915 ) ;
#18579=CARTESIAN_POINT ( 'NONE',  ( -85.40000000000000568, -33.58124999877097139, 98.26794919243111792 ) ) ;
#18590=CARTESIAN_POINT ( 'NONE',  ( -80.90000000000000568, -33.74606250001229313, 97.40192378864668399 ) ) ;
#18600=EDGE_CURVE ( 'NONE', #6642, #6725, #8325, .T. ) ;
#18602=( BOUNDED_CURVE ( )  B_SPLINE_CURVE ( 2, ( #15483, #12164, #10887, #12356, #18324, #7767, #13619, #262, #15094, #13720, #454, #1803, #2095, #6309, #5037, #16661, #1998, #3368, #17046, #3459, #10789, #9130, #361, #15185, #12263, #5132, #6505, #7861, #647, #6217, #8056, #6596, #18228, #12544, #16855, #3560, #18515, #10979, #18417, #15385, #14011, #11077, #1709, #3265, #9320, #4942, #4844, #7955, #16948, #9418, #9519, #9221, #18131, #15284, #7664, #4751, #10695, #16750, #1899, #13909, #13813, #6403, #546, #12450, #740, #9812, #11370, #10008, #8250, #14200, #2286, #17438, #3657, #8343, #1028, #9716, #6696, #12746, #6799, #15964, #5523, #12640, #13029, #6890, #18614, #18713, #14389, #837, #19001, #2571, #14104, #8533, #15774, #14482, #5336, #5621, #11273, #5231, #1114, #17337, #11180, #6980, #17242, #11567, #7071, #17144, #9623, #2382, #15584, #3846, #2194, #14299, #5433, #3947, #9912, #935, #12840, #8152, #15680, #18808, #15875, #12932, #3750, #2479, #8437, #18902, #11471, #4049, #1215, #216, #10650, #6268, #17728, #414, #8727 ),
 .UNSPECIFIED., .F., .F. ) 
 B_SPLINE_CURVE_WITH_KNOTS ( ( 3, 2, 2, 2, 2, 2, 2, 2, 2, 2, 2, 2, 2, 2, 2, 2, 2, 2, 2, 2, 2, 2, 2, 2, 2, 2, 2, 2, 2, 2, 2, 2, 2, 2, 2, 2, 2, 2, 2, 2, 2, 2, 2, 2, 2, 2, 2, 2, 2, 2, 2, 2, 2, 2, 2, 2, 2, 2, 2, 2, 2, 2, 2, 2, 2, 2, 2, 3 ),
 ( 0.000000000000000000, 0.01500076810536658638, 0.03000153621073317275, 0.04500230431609975740, 0.06000307242146634551, 0.07500384052683294056, 0.09000460863219951479, 0.1050053767375661029, 0.1200061448429326910, 0.1350069129482992791, 0.1500076810536658811, 0.1650084491590324554, 0.1800092172643990296, 0.1950099853697656316, 0.2100107534751322058, 0.2250115215804988078, 0.2400122896858653820, 0.2550130577912319563, 0.2700138258965985583, 0.2850145940019651603, 0.3000153621073317622, 0.3150161302126983087, 0.3300168983180649107, 0.3450176664234314572, 0.3600184345287980592, 0.3750192026341646612, 0.3900199707395312632, 0.4050207388448978096, 0.4200215069502644116, 0.4350222750556310136, 0.4500230431609976156, 0.4650238112663642176, 0.4800245793717307641, 0.4950253474770973106, 0.5100261155824639125, 0.5250268836878305700, 0.5400276517931971165, 0.5550284198985636630, 0.5700291880039303205, 0.5850299561092968670, 0.6000307242146635245, 0.6150314923200299599, 0.6300322604253966174, 0.6450330285307631639, 0.6600337966361298214, 0.6750345647414963679, 0.6900353328468629144, 0.7050361009522295719, 0.7200368690575961184, 0.7350376371629627759, 0.7500384052683293223, 0.7650391733736959798, 0.7800399414790625263, 0.7950407095844291838, 0.8100414776897956193, 0.8250422457951621658, 0.8400430139005288233, 0.8550437820058953697, 0.8700445501112620272, 0.8850453182166285737, 0.9000460863219952312, 0.9150468544273617777, 0.9300476225327284352, 0.9450483906380949817, 0.9600491587434615282, 0.9750499268488280746, 0.9900506949541946211, 1.000000000000000000 ),
 .UNSPECIFIED. ) 
 CURVE ( )  GEOMETRIC_REPRESENTATION_ITEM ( )  RATIONAL_B_SPLINE_CURVE ( ( 1.000000000000000000, 0.8660254037844387076, 1.000000000000000000, 0.8660254037844387076, 1.000000000000000000, 0.8660254037844387076, 1.000000000000000000, 0.8660254037844387076, 1.000000000000000000, 0.8660254037844387076, 1.000000000000000000, 0.8660254037844387076, 1.000000000000000000, 0.8660254037844387076, 1.000000000000000000, 0.8660254037844387076, 1.000000000000000000, 0.8660254037844387076, 1.000000000000000000, 0.8660254037844387076, 1.000000000000000000, 0.8660254037844387076, 1.000000000000000000, 0.8660254037844387076, 1.000000000000000000, 0.8660254037844387076, 1.000000000000000000, 0.8660254037844387076, 1.000000000000000000, 0.8660254037844387076, 1.000000000000000000, 0.8660254037844387076, 1.000000000000000000, 0.8660254037844387076, 1.000000000000000000, 0.8660254037844387076, 1.000000000000000000, 0.8660254037844387076, 1.000000000000000000, 0.8660254037844387076, 1.000000000000000000, 0.8660254037844387076, 1.000000000000000000, 0.8660254037844387076, 1.000000000000000000, 0.8660254037844387076, 1.000000000000000000, 0.8660254037844387076, 1.000000000000000000, 0.8660254037844387076, 1.000000000000000000, 0.8660254037844387076, 1.000000000000000000, 0.8660254037844387076, 1.000000000000000000, 0.8660254037844387076, 1.000000000000000000, 0.8660254037844387076, 1.000000000000000000, 0.8660254037844387076, 1.000000000000000000, 0.8660254037844387076, 1.000000000000000000, 0.8660254037844387076, 1.000000000000000000, 0.8660254037844387076, 1.000000000000000000, 0.8660254037844387076, 1.000000000000000000, 0.8660254037844387076, 1.000000000000000000, 0.8660254037844387076, 1.000000000000000000, 0.8660254037844387076, 1.000000000000000000, 0.8660254037844387076, 1.000000000000000000, 0.8660254037844387076, 1.000000000000000000, 0.8660254037844387076, 1.000000000000000000, 0.8660254037844387076, 1.000000000000000000, 0.8660254037844387076, 1.000000000000000000, 0.8660254037844387076, 1.000000000000000000, 0.8660254037844387076, 1.000000000000000000, 0.8660254037844387076, 1.000000000000000000, 0.8660254037844387076, 1.000000000000000000, 0.8660254037844387076, 1.000000000000000000, 0.8660254037844387076, 1.000000000000000000, 0.8660254037844387076, 1.000000000000000000, 0.8660254037844387076, 1.000000000000000000, 0.8660254037844387076, 1.000000000000000000, 0.8660254037844387076, 1.000000000000000000, 0.8660254037844387076, 1.000000000000000000, 0.8660254037844387076, 1.000000000000000000, 0.8660254037844387076, 1.000000000000000000, 0.8660254037844387076, 1.000000000000000000, 0.8660254037844387076, 1.000000000000000000, 0.8660254037844387076, 1.000000000000000000, 0.8660254037844387076, 1.000000000000000000, 0.8660254037844387076, 1.000000000000000000, 0.8660254037844387076, 1.000000000000000000, 0.8660254037844387076, 1.000000000000000000, 0.8660254037844387076, 1.000000000000000000, 0.8660254037844387076, 1.000000000000000000, 0.8660254037844387076, 1.000000000000000000, 0.8660254037844387076, 1.000000000000000000, 0.9111409417988175496, 0.9401539645359766606 ) ) 
 REPRESENTATION_ITEM ( '' )  );
#18605=CARTESIAN_POINT ( 'NONE',  ( -81.02178482187500208, -34.00312499938548427, 97.61286128772489690 ) ) ;
#18611=CARTESIAN_POINT ( 'NONE',  ( -82.40000000000000568, -34.78124999877096712, 102.9999999999999858 ) ) ;
#18614=CARTESIAN_POINT ( 'NONE',  ( -85.15643035625001289, -33.40312499938548285, 99.99999999999998579 ) ) ;
#18624=CARTESIAN_POINT ( 'NONE',  ( -82.39999999999999147, -34.16250000000000142, 96.53589838486223584 ) ) ;
#18634=CARTESIAN_POINT ( 'NONE',  ( -83.90000000000000568, -34.97268749875867400, 97.40192378864668399 ) ) ;
#18651=CARTESIAN_POINT ( 'NONE',  ( -79.64356964375001269, -33.55312499938548854, 101.5914258081833879 ) ) ;
#18663=CARTESIAN_POINT ( 'NONE',  ( -80.90000000000000568, -32.34374999877096712, 97.40192378864668399 ) ) ;
#18664=CARTESIAN_POINT ( 'NONE',  ( -79.39999999999999147, -34.63124999877096855, 98.26794919243110371 ) ) ;
#18677=CARTESIAN_POINT ( 'NONE',  ( -83.77821517812500929, -31.86562499938548498, 102.3871387122750889 ) ) ;
#18692=CARTESIAN_POINT ( 'NONE',  ( -79.39999999999999147, -30.71250000000000568, 101.7320508075688537 ) ) ;
#18695=EDGE_CURVE ( 'NONE', #15015, #17250, #8068, .T. ) ;
#18704=CARTESIAN_POINT ( 'NONE',  ( -85.15643035624999868, -32.91562499938549280, 101.5914258081833879 ) ) ;
#18708=CARTESIAN_POINT ( 'NONE',  ( -79.64356964375001269, -33.02812499938548285, 98.40857419181659793 ) ) ;
#18713=CARTESIAN_POINT ( 'NONE',  ( -85.15643035625001289, -33.44062499938548427, 98.40857419181659793 ) ) ;
#18721=ORIENTED_EDGE ( 'NONE', *, *, #14293, .T. ) ;
#18724=CARTESIAN_POINT ( 'NONE',  ( -79.39999999999999147, -32.92500000000000426, 99.99999999999998579 ) ) ;
#18728=ORIENTED_EDGE ( 'NONE', *, *, #18695, .F. ) ;
#18732=LINE ( 'NONE', #3868, #4528 ) ;
#18733=CARTESIAN_POINT ( 'NONE',  ( -82.39999999999999147, -30.33356250001229171, 103.4641016151377499 ) ) ;
#18749=CARTESIAN_POINT ( 'NONE',  ( -85.15643035624999868, -32.80312499938548854, 101.5914258081833879 ) ) ;
#18753=CARTESIAN_POINT ( 'NONE',  ( -82.40000000000000568, -30.95624999877097139, 96.99999999999998579 ) ) ;
#18759=CARTESIAN_POINT ( 'NONE',  ( -85.40000000000000568, -32.23124999877096997, 98.26794919243111792 ) ) ;
#18760=CARTESIAN_POINT ( 'NONE',  ( -79.64356964374999848, -31.82812499938548356, 99.99999999999998579 ) ) ;
#18764=ORIENTED_EDGE ( 'NONE', *, *, #2182, .T. ) ;
#18768=( BOUNDED_CURVE ( )  B_SPLINE_CURVE ( 2, ( #1571, #6257, #12110, #13475, #12203, #15039, #8789, #19253, #14745 ),
 .UNSPECIFIED., .F., .F. ) 
 B_SPLINE_CURVE_WITH_KNOTS ( ( 3, 2, 2, 2, 3 ),
 ( 0.6875000000000000000, 0.6944444444444444198, 0.7083333333333333703, 0.7222222222222222099, 0.7291666666666666297 ),
 .UNSPECIFIED. ) 
 CURVE ( )  GEOMETRIC_REPRESENTATION_ITEM ( )  RATIONAL_B_SPLINE_CURVE ( ( 0.9330127018922194093, 0.9330127018922194093, 1.000000000000000000, 0.8660254037844387076, 1.000000000000000000, 0.8660254037844387076, 1.000000000000000000, 0.9330127018922198534, 0.9330127018922192983 ) ) 
 REPRESENTATION_ITEM ( '' )  );
#18770=CARTESIAN_POINT ( 'NONE',  ( -83.43214152715523824, -35.00000000000000000, 97.15572402832313514 ) ) ;
#18771=CARTESIAN_POINT ( 'NONE',  ( -79.64356964374998427, -31.22812499938548569, 98.40857419181659793 ) ) ;
#18775=CARTESIAN_POINT ( 'NONE',  ( -79.39999999999999147, -33.76874999877097139, 99.99999999999998579 ) ) ;
#18781=CARTESIAN_POINT ( 'NONE',  ( -80.90000000000000568, -30.75000000000000355, 102.5980762113533018 ) ) ;
#18785=CARTESIAN_POINT ( 'NONE',  ( -82.40000000000001990, -33.26250000000000284, 97.00000000000000000 ) ) ;
#18787=CARTESIAN_POINT ( 'NONE',  ( -82.39999999999999147, -31.23750000000000071, 102.9999999999999858 ) ) ;
#18796=CARTESIAN_POINT ( 'NONE',  ( -81.02178482187500208, -33.70312499938548711, 102.3871387122750889 ) ) ;
#18800=CARTESIAN_POINT ( 'NONE',  ( -82.65380294351676582, -34.99990492518305274, 97.01075526832239859 ) ) ;
#18801=CARTESIAN_POINT ( 'NONE',  ( -79.64356964374999848, -34.86562499938548143, 99.99999999999998579 ) ) ;
#18808=CARTESIAN_POINT ( 'NONE',  ( -85.15643035625001289, -34.71562499938548285, 101.5914258081833879 ) ) ;
#18821=CARTESIAN_POINT ( 'NONE',  ( -83.90000000000000568, -34.57500000000000284, 97.40192378864668399 ) ) ;
#18830=CARTESIAN_POINT ( 'NONE',  ( -82.39999999999999147, -31.00856250001228887, 96.53589838486223584 ) ) ;
#18831=( BOUNDED_CURVE ( )  B_SPLINE_CURVE ( 2, ( #10554, #8701, #4306, #5773, #1187, #11632, #16417, #13282, #2739 ),
 .UNSPECIFIED., .F., .F. ) 
 B_SPLINE_CURVE_WITH_KNOTS ( ( 3, 2, 2, 2, 3 ),
 ( 0.2291666666666666574, 0.2361111111111111049, 0.2500000000000000000, 0.2638888888888888951, 0.2708333333333333703 ),
 .UNSPECIFIED. ) 
 CURVE ( )  GEOMETRIC_REPRESENTATION_ITEM ( )  RATIONAL_B_SPLINE_CURVE ( ( 0.9330127018922194093, 0.9330127018922194093, 1.000000000000000000, 0.8660254037844387076, 1.000000000000000000, 0.8660254037844387076, 1.000000000000000000, 0.9330127018922190762, 0.9330127018922194093 ) ) 
 REPRESENTATION_ITEM ( '' )  );
#18832=DIRECTION ( 'NONE',  ( 0.000000000000000000, 0.000000000000000000, -1.000000000000000000 ) ) ;
#18845=CARTESIAN_POINT ( 'NONE',  ( -84.51154815724953551, -35.14114861271051637, 98.22820072003833047 ) ) ;
#18857=CARTESIAN_POINT ( 'NONE',  ( -85.40000000000000568, -35.30624999877096570, 101.7320508075688679 ) ) ;
#18858=CARTESIAN_POINT ( 'NONE',  ( -81.02178482187500208, -30.40312499938548640, 97.61286128772489690 ) ) ;
#18867=CARTESIAN_POINT ( 'NONE',  ( -84.13153929418699306, -35.00000000000000000, 97.51867099968119135 ) ) ;
#18868=CARTESIAN_POINT ( 'NONE',  ( -83.77821517812500929, -30.51562499938548711, 102.3871387122750889 ) ) ;
#18879=CARTESIAN_POINT ( 'NONE',  ( -82.39999999999999147, -32.36250000000000426, 96.53589838486223584 ) ) ;
#18887=ORIENTED_EDGE ( 'NONE', *, *, #2229, .F. ) ;
#18894=CARTESIAN_POINT ( 'NONE',  ( -79.64356964375001269, -32.69062499938548427, 98.40857419181659793 ) ) ;
#18897=CARTESIAN_POINT ( 'NONE',  ( -82.39999999999999147, -34.30312499938548143, 96.81714838363319586 ) ) ;
#18902=CARTESIAN_POINT ( 'NONE',  ( -79.64356964374998427, -34.94062499938548427, 98.40857419181659793 ) ) ;
#18914=CARTESIAN_POINT ( 'NONE',  ( -83.90000000000000568, -33.97500000000000853, 102.5980762113533018 ) ) ;
#18927=CARTESIAN_POINT ( 'NONE',  ( -85.40000000000000568, -33.56250000000000000, 101.7320508075688821 ) ) ;
#18937=CARTESIAN_POINT ( 'NONE',  ( -82.40000000000000568, -31.63124999877096855, 102.9999999999999858 ) ) ;
#18950=CARTESIAN_POINT ( 'NONE',  ( -85.40000000000000568, -30.39768749875867826, 99.99999999999998579 ) ) ;
#18951=AXIS2_PLACEMENT_3D ( 'NONE', #6662, #11137, #10755 ) ;
#18952=CARTESIAN_POINT ( 'NONE',  ( -79.64356964375001269, -30.51562499938548711, 101.5914258081833879 ) ) ;
#18965=CARTESIAN_POINT ( 'NONE',  ( -79.64356964374999848, -31.71562499938548285, 99.99999999999998579 ) ) ;
#18976=CARTESIAN_POINT ( 'NONE',  ( -79.39999999999999147, -31.57499999999999929, 99.99999999999998579 ) ) ;
#18989=CARTESIAN_POINT ( 'NONE',  ( -81.59615242270662350, -33.41115380933863577, 102.9999999999999858 ) ) ;
#18991=CARTESIAN_POINT ( 'NONE',  ( -81.02178482187500208, -34.15312499938548285, 102.3871387122750889 ) ) ;
#18992=DIRECTION ( 'NONE',  ( 0.7660487055105749121, 0.000000000000000000, 0.6427825299318367103 ) ) ;
#18995=CARTESIAN_POINT ( 'NONE',  ( -85.15643035625001289, -34.64062499938548711, 99.99999999999998579 ) ) ;
#18998=AXIS2_PLACEMENT_3D ( 'NONE', #13392, #10652, #10748 ) ;
#19001=CARTESIAN_POINT ( 'NONE',  ( -81.02178482187500208, -33.55312499938548854, 97.61286128772489690 ) ) ;
#19011=CARTESIAN_POINT ( 'NONE',  ( -80.90000000000000568, -33.30000000000000426, 97.40192378864668399 ) ) ;
#19042=CARTESIAN_POINT ( 'NONE',  ( -83.90000000000000568, -34.06874999877096855, 97.40192378864668399 ) ) ;
#19043=CARTESIAN_POINT ( 'NONE',  ( -85.15643035624999868, -31.64062499938548356, 98.40857419181659793 ) ) ;
#19057=CARTESIAN_POINT ( 'NONE',  ( -80.90000000000000568, -35.04374999877096997, 97.40192378864668399 ) ) ;
#19058=CARTESIAN_POINT ( 'NONE',  ( -85.15643035625001289, -31.90312499938548285, 101.5914258081833879 ) ) ;
#19059=ORIENTED_EDGE ( 'NONE', *, *, #2950, .F. ) ;
#19060=VERTEX_POINT ( 'NONE', #8940 ) ;
#19069=CARTESIAN_POINT ( 'NONE',  ( -79.39999999999999147, -32.51250000000000284, 101.7320508075688537 ) ) ;
#19071=LINE ( 'NONE', #13006, #14600 ) ;
#19072=CARTESIAN_POINT ( 'NONE',  ( -84.69814171518287083, -35.32864829504264748, 98.07164716482272127 ) ) ;
#19080=CARTESIAN_POINT ( 'NONE',  ( -83.77821517812500929, -31.11562499938548498, 97.61286128772489690 ) ) ;
#19082=ADVANCED_FACE ( 'NONE', ( #17941 ), #19215, .T. ) ;
#19084=ORIENTED_EDGE ( 'NONE', *, *, #2361, .T. ) ;
#19086=CARTESIAN_POINT ( 'NONE',  ( -85.15643035624999868, -34.22812499938547859, 98.40857419181659793 ) ) ;
#19087=CARTESIAN_POINT ( 'NONE',  ( -82.40000000000000568, -30.00000000000000355, 96.99999999999998579 ) ) ;
#19089=LINE ( 'NONE', #1211, #4001 ) ;
#19110=CARTESIAN_POINT ( 'NONE',  ( -83.90000000000000568, -33.52106250001229171, 102.5980762113533018 ) ) ;
#19113=CARTESIAN_POINT ( 'NONE',  ( -79.64356964375001269, -32.57812499938548001, 98.40857419181659793 ) ) ;
#19127=ORIENTED_EDGE ( 'NONE', *, *, #18695, .T. ) ;
#19130=ORIENTED_EDGE ( 'NONE', *, *, #16871, .T. ) ;
#19137=CARTESIAN_POINT ( 'NONE',  ( -85.40000000000000568, -30.43518749875867968, 98.26794919243111792 ) ) ;
#19138=CARTESIAN_POINT ( 'NONE',  ( -79.64356964374999848, -32.27812499938548996, 99.99999999999998579 ) ) ;
#19152=CARTESIAN_POINT ( 'NONE',  ( -79.64356964374998427, -33.55312499938548854, 101.5914258081833879 ) ) ;
#19154=VERTEX_POINT ( 'NONE', #19319 ) ;
#19164=CARTESIAN_POINT ( 'NONE',  ( -82.39999999999999147, -31.01249999999999929, 96.53589838486223584 ) ) ;
#19177=CARTESIAN_POINT ( 'NONE',  ( -85.15643035624999868, -30.17812499938548498, 98.40857419181659793 ) ) ;
#19183=CARTESIAN_POINT ( 'NONE',  ( -85.40000000000000568, -31.35000000000000142, 99.99999999999998579 ) ) ;
#19191=CARTESIAN_POINT ( 'NONE',  ( -80.90000000000000568, -30.60000000000000142, 97.40192378864668399 ) ) ;
#19209=CARTESIAN_POINT ( 'NONE',  ( -82.39999999999999147, -32.13356250001228887, 103.4641016151377499 ) ) ;
#19211=CARTESIAN_POINT ( 'NONE',  ( -83.77821517812500929, -32.76562499938548711, 102.3871387122750889 ) ) ;
#19215=CYLINDRICAL_SURFACE ( 'NONE', #9633, 3.000000000000002665 ) ;
#19220=CYLINDRICAL_SURFACE ( 'NONE', #17714, 3.000000000000002665 ) ;
#19236=CARTESIAN_POINT ( 'NONE',  ( -82.39999999999999147, -33.88124999877096855, 103.4641016151377499 ) ) ;
#19237=CARTESIAN_POINT ( 'NONE',  ( -82.39999999999999147, -34.64062499938548711, 103.1828516163667899 ) ) ;
#19249=CARTESIAN_POINT ( 'NONE',  ( -81.02178482187500208, -33.44062499938548427, 97.61286128772489690 ) ) ;
#19253=CARTESIAN_POINT ( 'NONE',  ( -81.59615242270662350, -34.31115380933863435, 102.9999999999999716 ) ) ;
#19261=CARTESIAN_POINT ( 'NONE',  ( -79.39999999999999147, -32.02500000000000568, 99.99999999999998579 ) ) ;
#19262=CARTESIAN_POINT ( 'NONE',  ( -79.39999999999999147, -32.38124999877096855, 98.26794919243110371 ) ) ;
#19264=DIRECTION ( 'NONE',  ( -0.000000000000000000, -1.000000000000000000, -0.000000000000000000 ) ) ;
#19265=CARTESIAN_POINT ( 'NONE',  ( -84.69814078818293979, -35.03295773984034867, 98.07164606005757435 ) ) ;
#19270=DIRECTION ( 'NONE',  ( 0.000000000000000000, 0.000000000000000000, 1.000000000000000000 ) ) ;
#19276=CARTESIAN_POINT ( 'NONE',  ( -83.77821517812500929, -32.01562499938548001, 97.61286128772489690 ) ) ;
#19284=CARTESIAN_POINT ( 'NONE',  ( -85.40000000000000568, -32.21249999999999858, 101.7320508075688679 ) ) ;
#19302=CARTESIAN_POINT ( 'NONE',  ( -82.40000000000000568, -50.00000000000000000, 99.99999999999998579 ) ) ;
#19311=CARTESIAN_POINT ( 'NONE',  ( -79.39999999999999147, -32.02106250001229881, 99.99999999999998579 ) ) ;
#19315=CARTESIAN_POINT ( 'NONE',  ( -85.15643035624999868, -31.07812499938548356, 98.40857419181659793 ) ) ;
#19319=CARTESIAN_POINT ( 'NONE',  ( -82.40000000000000568, -33.43124999877096570, 102.9999999999999858 ) ) ;
#19321=CARTESIAN_POINT ( 'NONE',  ( -83.90000000000000568, -30.77268749875868181, 102.5980762113533018 ) ) ;
#19351=COLOUR_RGB('Sky Blue',0.24,0.69,0.87);
#19352=FILL_AREA_STYLE_COLOUR('',#19351);
#19353=FILL_AREA_STYLE('',(#19352));
#19354=SURFACE_STYLE_FILL_AREA(#19353);
#19355=SURFACE_SIDE_STYLE('',(#19354));
#19356=SURFACE_STYLE_USAGE(.BOTH.,#19355);
#19357=PRESENTATION_STYLE_ASSIGNMENT((#19356));
ENDSEC;
END-ISO-10303-21;
